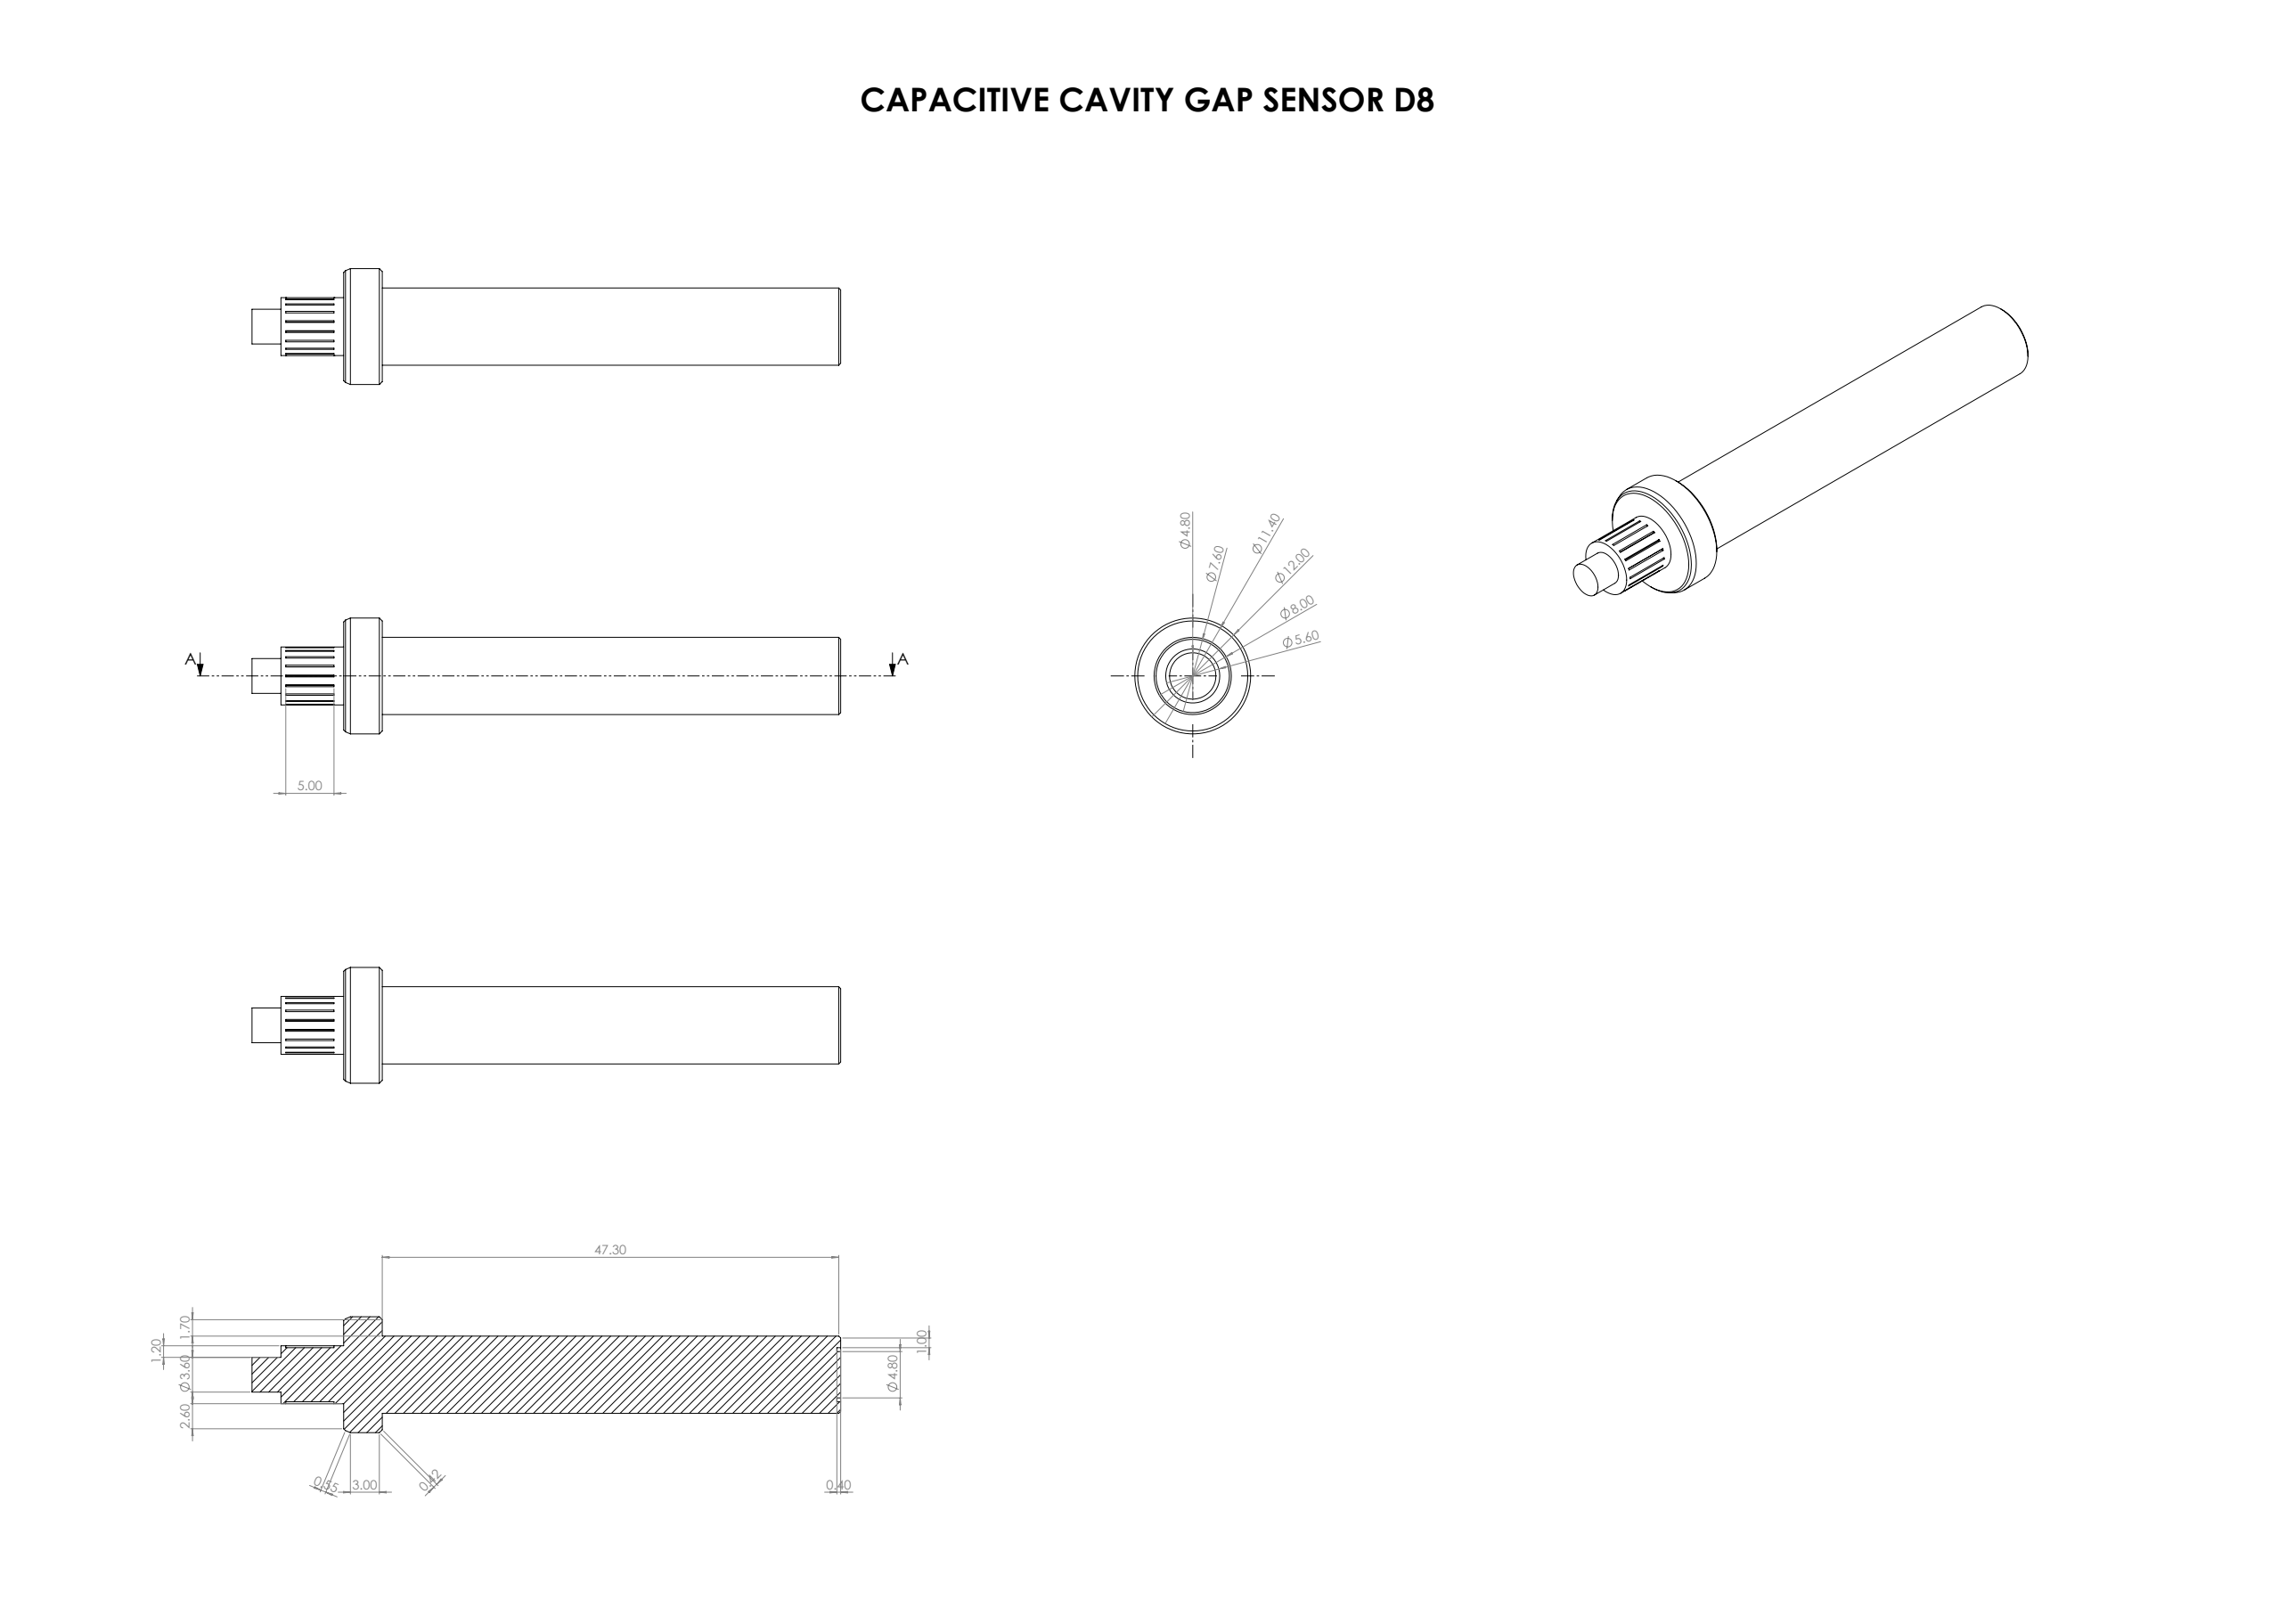
ISO-10303-21;
HEADER;
/* Generated by software containing ST-Developer
 * from STEP Tools, Inc. (www.steptools.com) 
 */

FILE_DESCRIPTION(
/* description */ (''),
/* implementation_level */ '2;1');

FILE_NAME(
/* name */ '07_Capacitive_Cavity_Gap_Sensor_D8.step',
/* time_stamp */ '2026-10-19T22:59:19-07:00',
/* author */ (''),
/* organization */ (''),
/* preprocessor_version */ 'ST-DEVELOPER v20.2',
/* originating_system */ 'Autodesk Translation Framework v15.15.0.0',
/* authorisation */ '');

FILE_SCHEMA (('AUTOMOTIVE_DESIGN { 1 0 10303 214 3 1 1 }'));
ENDSEC;

DATA;
#10=MECHANICAL_DESIGN_GEOMETRIC_PRESENTATION_REPRESENTATION('',(#919),#53650);
#887=SHAPE_REPRESENTATION_RELATIONSHIP('SRR','None',#53732,#903);
#903=ADVANCED_BREP_SHAPE_REPRESENTATION('',(#935),#53642);
#919=STYLED_ITEM('',(#53944),#935);
#935=MANIFOLD_SOLID_BREP('Gap Sensor',#23311);
#1038=CYLINDRICAL_SURFACE('',#24380,0.6);
#1039=CYLINDRICAL_SURFACE('',#24499,0.24);
#1040=CYLINDRICAL_SURFACE('',#24502,0.28);
#1041=CYLINDRICAL_SURFACE('',#24511,0.4);
#1042=CYLINDRICAL_SURFACE('',#24514,0.3);
#1043=CYLINDRICAL_SURFACE('',#24518,0.18);
#1388=FACE_BOUND('',#4169,.T.);
#1389=FACE_BOUND('',#4245,.T.);
#1390=FACE_BOUND('',#4247,.T.);
#1391=FACE_BOUND('',#4252,.T.);
#1392=FACE_BOUND('',#4254,.T.);
#1393=FACE_BOUND('',#4255,.T.);
#1394=FACE_BOUND('',#4256,.T.);
#1395=FACE_BOUND('',#4257,.T.);
#1396=FACE_BOUND('',#4258,.T.);
#1397=FACE_BOUND('',#4259,.T.);
#1398=FACE_BOUND('',#4260,.T.);
#1399=FACE_BOUND('',#4261,.T.);
#1400=FACE_BOUND('',#4262,.T.);
#1401=FACE_BOUND('',#4263,.T.);
#1402=FACE_BOUND('',#4264,.T.);
#1403=FACE_BOUND('',#4265,.T.);
#1404=FACE_BOUND('',#4266,.T.);
#1405=FACE_BOUND('',#4267,.T.);
#1406=FACE_BOUND('',#4268,.T.);
#1407=FACE_BOUND('',#4269,.T.);
#1408=FACE_BOUND('',#4270,.T.);
#1409=FACE_BOUND('',#4272,.T.);
#1676=PLANE('',#24387);
#1677=PLANE('',#24389);
#1678=PLANE('',#24390);
#1679=PLANE('',#24392);
#1680=PLANE('',#24393);
#1681=PLANE('',#24395);
#1682=PLANE('',#24396);
#1683=PLANE('',#24398);
#1684=PLANE('',#24399);
#1685=PLANE('',#24401);
#1686=PLANE('',#24402);
#1687=PLANE('',#24404);
#1688=PLANE('',#24405);
#1689=PLANE('',#24407);
#1690=PLANE('',#24408);
#1691=PLANE('',#24410);
#1692=PLANE('',#24411);
#1693=PLANE('',#24413);
#1694=PLANE('',#24414);
#1695=PLANE('',#24416);
#1696=PLANE('',#24417);
#1697=PLANE('',#24419);
#1698=PLANE('',#24420);
#1699=PLANE('',#24422);
#1700=PLANE('',#24423);
#1701=PLANE('',#24425);
#1702=PLANE('',#24426);
#1703=PLANE('',#24428);
#1704=PLANE('',#24429);
#1705=PLANE('',#24431);
#1706=PLANE('',#24432);
#1707=PLANE('',#24434);
#1708=PLANE('',#24435);
#1709=PLANE('',#24437);
#1710=PLANE('',#24438);
#1711=PLANE('',#24441);
#1712=PLANE('',#24442);
#1713=PLANE('',#24445);
#1714=PLANE('',#24446);
#1715=PLANE('',#24448);
#1716=PLANE('',#24449);
#1717=PLANE('',#24451);
#1718=PLANE('',#24452);
#1719=PLANE('',#24454);
#1720=PLANE('',#24455);
#1721=PLANE('',#24457);
#1722=PLANE('',#24458);
#1723=PLANE('',#24460);
#1724=PLANE('',#24461);
#1725=PLANE('',#24463);
#1726=PLANE('',#24464);
#1727=PLANE('',#24466);
#1728=PLANE('',#24467);
#1729=PLANE('',#24469);
#1730=PLANE('',#24470);
#1731=PLANE('',#24472);
#1732=PLANE('',#24473);
#1733=PLANE('',#24475);
#1734=PLANE('',#24476);
#1735=PLANE('',#24478);
#1736=PLANE('',#24479);
#1737=PLANE('',#24481);
#1738=PLANE('',#24482);
#1739=PLANE('',#24484);
#1740=PLANE('',#24485);
#1741=PLANE('',#24487);
#1742=PLANE('',#24488);
#1743=PLANE('',#24490);
#1744=PLANE('',#24491);
#1745=PLANE('',#24493);
#1746=PLANE('',#24494);
#1747=PLANE('',#24496);
#1748=PLANE('',#24497);
#1749=PLANE('',#24505);
#1750=PLANE('',#24506);
#1751=PLANE('',#24508);
#1752=PLANE('',#24512);
#1753=PLANE('',#24516);
#1754=PLANE('',#24520);
#2725=FACE_OUTER_BOUND('',#4164,.T.);
#2726=FACE_OUTER_BOUND('',#4165,.T.);
#2727=FACE_OUTER_BOUND('',#4166,.T.);
#2728=FACE_OUTER_BOUND('',#4167,.T.);
#2729=FACE_OUTER_BOUND('',#4168,.T.);
#2730=FACE_OUTER_BOUND('',#4170,.T.);
#2731=FACE_OUTER_BOUND('',#4171,.T.);
#2732=FACE_OUTER_BOUND('',#4172,.T.);
#2733=FACE_OUTER_BOUND('',#4173,.T.);
#2734=FACE_OUTER_BOUND('',#4174,.T.);
#2735=FACE_OUTER_BOUND('',#4175,.T.);
#2736=FACE_OUTER_BOUND('',#4176,.T.);
#2737=FACE_OUTER_BOUND('',#4177,.T.);
#2738=FACE_OUTER_BOUND('',#4178,.T.);
#2739=FACE_OUTER_BOUND('',#4179,.T.);
#2740=FACE_OUTER_BOUND('',#4180,.T.);
#2741=FACE_OUTER_BOUND('',#4181,.T.);
#2742=FACE_OUTER_BOUND('',#4182,.T.);
#2743=FACE_OUTER_BOUND('',#4183,.T.);
#2744=FACE_OUTER_BOUND('',#4184,.T.);
#2745=FACE_OUTER_BOUND('',#4185,.T.);
#2746=FACE_OUTER_BOUND('',#4186,.T.);
#2747=FACE_OUTER_BOUND('',#4187,.T.);
#2748=FACE_OUTER_BOUND('',#4188,.T.);
#2749=FACE_OUTER_BOUND('',#4189,.T.);
#2750=FACE_OUTER_BOUND('',#4190,.T.);
#2751=FACE_OUTER_BOUND('',#4191,.T.);
#2752=FACE_OUTER_BOUND('',#4192,.T.);
#2753=FACE_OUTER_BOUND('',#4193,.T.);
#2754=FACE_OUTER_BOUND('',#4194,.T.);
#2755=FACE_OUTER_BOUND('',#4195,.T.);
#2756=FACE_OUTER_BOUND('',#4196,.T.);
#2757=FACE_OUTER_BOUND('',#4197,.T.);
#2758=FACE_OUTER_BOUND('',#4198,.T.);
#2759=FACE_OUTER_BOUND('',#4199,.T.);
#2760=FACE_OUTER_BOUND('',#4200,.T.);
#2761=FACE_OUTER_BOUND('',#4201,.T.);
#2762=FACE_OUTER_BOUND('',#4202,.T.);
#2763=FACE_OUTER_BOUND('',#4203,.T.);
#2764=FACE_OUTER_BOUND('',#4204,.T.);
#2765=FACE_OUTER_BOUND('',#4205,.T.);
#2766=FACE_OUTER_BOUND('',#4206,.T.);
#2767=FACE_OUTER_BOUND('',#4207,.T.);
#2768=FACE_OUTER_BOUND('',#4208,.T.);
#2769=FACE_OUTER_BOUND('',#4209,.T.);
#2770=FACE_OUTER_BOUND('',#4210,.T.);
#2771=FACE_OUTER_BOUND('',#4211,.T.);
#2772=FACE_OUTER_BOUND('',#4212,.T.);
#2773=FACE_OUTER_BOUND('',#4213,.T.);
#2774=FACE_OUTER_BOUND('',#4214,.T.);
#2775=FACE_OUTER_BOUND('',#4215,.T.);
#2776=FACE_OUTER_BOUND('',#4216,.T.);
#2777=FACE_OUTER_BOUND('',#4217,.T.);
#2778=FACE_OUTER_BOUND('',#4218,.T.);
#2779=FACE_OUTER_BOUND('',#4219,.T.);
#2780=FACE_OUTER_BOUND('',#4220,.T.);
#2781=FACE_OUTER_BOUND('',#4221,.T.);
#2782=FACE_OUTER_BOUND('',#4222,.T.);
#2783=FACE_OUTER_BOUND('',#4223,.T.);
#2784=FACE_OUTER_BOUND('',#4224,.T.);
#2785=FACE_OUTER_BOUND('',#4225,.T.);
#2786=FACE_OUTER_BOUND('',#4226,.T.);
#2787=FACE_OUTER_BOUND('',#4227,.T.);
#2788=FACE_OUTER_BOUND('',#4228,.T.);
#2789=FACE_OUTER_BOUND('',#4229,.T.);
#2790=FACE_OUTER_BOUND('',#4230,.T.);
#2791=FACE_OUTER_BOUND('',#4231,.T.);
#2792=FACE_OUTER_BOUND('',#4232,.T.);
#2793=FACE_OUTER_BOUND('',#4233,.T.);
#2794=FACE_OUTER_BOUND('',#4234,.T.);
#2795=FACE_OUTER_BOUND('',#4235,.T.);
#2796=FACE_OUTER_BOUND('',#4236,.T.);
#2797=FACE_OUTER_BOUND('',#4237,.T.);
#2798=FACE_OUTER_BOUND('',#4238,.T.);
#2799=FACE_OUTER_BOUND('',#4239,.T.);
#2800=FACE_OUTER_BOUND('',#4240,.T.);
#2801=FACE_OUTER_BOUND('',#4241,.T.);
#2802=FACE_OUTER_BOUND('',#4242,.T.);
#2803=FACE_OUTER_BOUND('',#4243,.T.);
#2804=FACE_OUTER_BOUND('',#4244,.T.);
#2805=FACE_OUTER_BOUND('',#4246,.T.);
#2806=FACE_OUTER_BOUND('',#4248,.T.);
#2807=FACE_OUTER_BOUND('',#4249,.T.);
#2808=FACE_OUTER_BOUND('',#4250,.T.);
#2809=FACE_OUTER_BOUND('',#4251,.T.);
#2810=FACE_OUTER_BOUND('',#4253,.T.);
#2811=FACE_OUTER_BOUND('',#4271,.T.);
#2812=FACE_OUTER_BOUND('',#4273,.T.);
#2813=FACE_OUTER_BOUND('',#4274,.T.);
#4164=EDGE_LOOP('',(#17227,#17228,#17229,#17230,#17231,#17232));
#4165=EDGE_LOOP('',(#17233,#17234,#17235,#17236,#17237,#17238));
#4166=EDGE_LOOP('',(#17239,#17240,#17241,#17242,#17243));
#4167=EDGE_LOOP('',(#17244,#17245,#17246,#17247,#17248));
#4168=EDGE_LOOP('',(#17249));
#4169=EDGE_LOOP('',(#17250));
#4170=EDGE_LOOP('',(#17251,#17252,#17253,#17254));
#4171=EDGE_LOOP('',(#17255,#17256,#17257));
#4172=EDGE_LOOP('',(#17258,#17259,#17260,#17261));
#4173=EDGE_LOOP('',(#17262,#17263,#17264));
#4174=EDGE_LOOP('',(#17265,#17266,#17267,#17268));
#4175=EDGE_LOOP('',(#17269,#17270,#17271));
#4176=EDGE_LOOP('',(#17272,#17273,#17274,#17275));
#4177=EDGE_LOOP('',(#17276,#17277,#17278));
#4178=EDGE_LOOP('',(#17279,#17280,#17281,#17282));
#4179=EDGE_LOOP('',(#17283,#17284,#17285));
#4180=EDGE_LOOP('',(#17286,#17287,#17288,#17289));
#4181=EDGE_LOOP('',(#17290,#17291,#17292));
#4182=EDGE_LOOP('',(#17293,#17294,#17295,#17296));
#4183=EDGE_LOOP('',(#17297,#17298,#17299));
#4184=EDGE_LOOP('',(#17300,#17301,#17302,#17303));
#4185=EDGE_LOOP('',(#17304,#17305,#17306));
#4186=EDGE_LOOP('',(#17307,#17308,#17309,#17310));
#4187=EDGE_LOOP('',(#17311,#17312,#17313));
#4188=EDGE_LOOP('',(#17314,#17315,#17316,#17317));
#4189=EDGE_LOOP('',(#17318,#17319,#17320));
#4190=EDGE_LOOP('',(#17321,#17322,#17323,#17324));
#4191=EDGE_LOOP('',(#17325,#17326,#17327));
#4192=EDGE_LOOP('',(#17328,#17329,#17330,#17331));
#4193=EDGE_LOOP('',(#17332,#17333,#17334));
#4194=EDGE_LOOP('',(#17335,#17336,#17337,#17338));
#4195=EDGE_LOOP('',(#17339,#17340,#17341));
#4196=EDGE_LOOP('',(#17342,#17343,#17344,#17345));
#4197=EDGE_LOOP('',(#17346,#17347,#17348));
#4198=EDGE_LOOP('',(#17349,#17350,#17351,#17352));
#4199=EDGE_LOOP('',(#17353,#17354,#17355));
#4200=EDGE_LOOP('',(#17356,#17357,#17358,#17359));
#4201=EDGE_LOOP('',(#17360,#17361,#17362));
#4202=EDGE_LOOP('',(#17363,#17364,#17365,#17366));
#4203=EDGE_LOOP('',(#17367,#17368,#17369,#17370));
#4204=EDGE_LOOP('',(#17371,#17372,#17373,#17374));
#4205=EDGE_LOOP('',(#17375,#17376,#17377,#17378));
#4206=EDGE_LOOP('',(#17379,#17380,#17381,#17382));
#4207=EDGE_LOOP('',(#17383,#17384,#17385));
#4208=EDGE_LOOP('',(#17386,#17387,#17388,#17389));
#4209=EDGE_LOOP('',(#17390,#17391,#17392));
#4210=EDGE_LOOP('',(#17393,#17394,#17395,#17396));
#4211=EDGE_LOOP('',(#17397,#17398,#17399));
#4212=EDGE_LOOP('',(#17400,#17401,#17402,#17403));
#4213=EDGE_LOOP('',(#17404,#17405,#17406));
#4214=EDGE_LOOP('',(#17407,#17408,#17409,#17410));
#4215=EDGE_LOOP('',(#17411,#17412,#17413));
#4216=EDGE_LOOP('',(#17414,#17415,#17416,#17417));
#4217=EDGE_LOOP('',(#17418,#17419,#17420));
#4218=EDGE_LOOP('',(#17421,#17422,#17423,#17424));
#4219=EDGE_LOOP('',(#17425,#17426,#17427));
#4220=EDGE_LOOP('',(#17428,#17429,#17430,#17431));
#4221=EDGE_LOOP('',(#17432,#17433,#17434));
#4222=EDGE_LOOP('',(#17435,#17436,#17437,#17438));
#4223=EDGE_LOOP('',(#17439,#17440,#17441));
#4224=EDGE_LOOP('',(#17442,#17443,#17444,#17445));
#4225=EDGE_LOOP('',(#17446,#17447,#17448));
#4226=EDGE_LOOP('',(#17449,#17450,#17451,#17452));
#4227=EDGE_LOOP('',(#17453,#17454,#17455));
#4228=EDGE_LOOP('',(#17456,#17457,#17458,#17459));
#4229=EDGE_LOOP('',(#17460,#17461,#17462));
#4230=EDGE_LOOP('',(#17463,#17464,#17465,#17466));
#4231=EDGE_LOOP('',(#17467,#17468,#17469));
#4232=EDGE_LOOP('',(#17470,#17471,#17472,#17473));
#4233=EDGE_LOOP('',(#17474,#17475,#17476));
#4234=EDGE_LOOP('',(#17477,#17478,#17479,#17480));
#4235=EDGE_LOOP('',(#17481,#17482,#17483));
#4236=EDGE_LOOP('',(#17484,#17485,#17486,#17487));
#4237=EDGE_LOOP('',(#17488,#17489,#17490));
#4238=EDGE_LOOP('',(#17491,#17492,#17493,#17494));
#4239=EDGE_LOOP('',(#17495,#17496,#17497));
#4240=EDGE_LOOP('',(#17498,#17499,#17500,#17501));
#4241=EDGE_LOOP('',(#17502,#17503,#17504));
#4242=EDGE_LOOP('',(#17505,#17506,#17507,#17508));
#4243=EDGE_LOOP('',(#17509,#17510,#17511,#17512));
#4244=EDGE_LOOP('',(#17513));
#4245=EDGE_LOOP('',(#17514));
#4246=EDGE_LOOP('',(#17515));
#4247=EDGE_LOOP('',(#17516));
#4248=EDGE_LOOP('',(#17517));
#4249=EDGE_LOOP('',(#17518,#17519,#17520,#17521));
#4250=EDGE_LOOP('',(#17522,#17523,#17524,#17525));
#4251=EDGE_LOOP('',(#17526));
#4252=EDGE_LOOP('',(#17527));
#4253=EDGE_LOOP('',(#17528,#17529,#17530,#17531,#17532,#17533,#17534,#17535,
#17536,#17537,#17538,#17539));
#4254=EDGE_LOOP('',(#17540,#17541,#17542,#17543));
#4255=EDGE_LOOP('',(#17544,#17545,#17546,#17547));
#4256=EDGE_LOOP('',(#17548,#17549,#17550,#17551));
#4257=EDGE_LOOP('',(#17552,#17553,#17554,#17555));
#4258=EDGE_LOOP('',(#17556,#17557,#17558,#17559));
#4259=EDGE_LOOP('',(#17560,#17561,#17562,#17563));
#4260=EDGE_LOOP('',(#17564,#17565,#17566,#17567));
#4261=EDGE_LOOP('',(#17568,#17569,#17570,#17571));
#4262=EDGE_LOOP('',(#17572,#17573,#17574,#17575));
#4263=EDGE_LOOP('',(#17576,#17577,#17578,#17579));
#4264=EDGE_LOOP('',(#17580,#17581,#17582,#17583));
#4265=EDGE_LOOP('',(#17584,#17585,#17586,#17587));
#4266=EDGE_LOOP('',(#17588,#17589,#17590,#17591));
#4267=EDGE_LOOP('',(#17592,#17593,#17594,#17595));
#4268=EDGE_LOOP('',(#17596,#17597,#17598,#17599));
#4269=EDGE_LOOP('',(#17600,#17601,#17602,#17603));
#4270=EDGE_LOOP('',(#17604,#17605,#17606,#17607));
#4271=EDGE_LOOP('',(#17608));
#4272=EDGE_LOOP('',(#17609));
#4273=EDGE_LOOP('',(#17610,#17611,#17612,#17613));
#4274=EDGE_LOOP('',(#17614));
#5445=CIRCLE('',#24376,0.578786796564404);
#5446=CIRCLE('',#24377,0.578786796564404);
#5447=CIRCLE('',#24378,0.6);
#5448=CIRCLE('',#24379,0.6);
#5449=CIRCLE('',#24381,0.6);
#5450=CIRCLE('',#24382,0.6);
#5451=CIRCLE('',#24384,0.56);
#5452=CIRCLE('',#24386,0.57);
#5453=CIRCLE('',#24388,0.4);
#5454=CIRCLE('',#24391,0.3);
#5455=CIRCLE('',#24394,0.3);
#5456=CIRCLE('',#24397,0.3);
#5457=CIRCLE('',#24400,0.3);
#5458=CIRCLE('',#24403,0.3);
#5459=CIRCLE('',#24406,0.3);
#5460=CIRCLE('',#24409,0.3);
#5461=CIRCLE('',#24412,0.3);
#5462=CIRCLE('',#24415,0.3);
#5463=CIRCLE('',#24418,0.3);
#5464=CIRCLE('',#24421,0.3);
#5465=CIRCLE('',#24424,0.3);
#5466=CIRCLE('',#24427,0.3);
#5467=CIRCLE('',#24430,0.3);
#5468=CIRCLE('',#24433,0.3);
#5469=CIRCLE('',#24436,0.3);
#5470=CIRCLE('',#24439,0.3);
#5471=CIRCLE('',#24440,0.3);
#5472=CIRCLE('',#24443,0.3);
#5473=CIRCLE('',#24444,0.3);
#5474=CIRCLE('',#24447,0.3);
#5475=CIRCLE('',#24450,0.3);
#5476=CIRCLE('',#24453,0.3);
#5477=CIRCLE('',#24456,0.3);
#5478=CIRCLE('',#24459,0.3);
#5479=CIRCLE('',#24462,0.3);
#5480=CIRCLE('',#24465,0.3);
#5481=CIRCLE('',#24468,0.3);
#5482=CIRCLE('',#24471,0.3);
#5483=CIRCLE('',#24474,0.3);
#5484=CIRCLE('',#24477,0.3);
#5485=CIRCLE('',#24480,0.3);
#5486=CIRCLE('',#24483,0.3);
#5487=CIRCLE('',#24486,0.3);
#5488=CIRCLE('',#24489,0.3);
#5489=CIRCLE('',#24492,0.3);
#5490=CIRCLE('',#24495,0.3);
#5491=CIRCLE('',#24498,0.3);
#5492=CIRCLE('',#24500,0.24);
#5493=CIRCLE('',#24501,0.24);
#5494=CIRCLE('',#24503,0.28);
#5495=CIRCLE('',#24504,0.28);
#5496=CIRCLE('',#24507,0.38);
#5497=CIRCLE('',#24510,0.4);
#5498=CIRCLE('',#24513,0.3);
#5499=CIRCLE('',#24515,0.3);
#5500=CIRCLE('',#24517,0.18);
#5501=CIRCLE('',#24519,0.18);
#6499=LINE('',#35561,#8344);
#6500=LINE('',#35567,#8345);
#6501=LINE('',#35574,#8346);
#6502=LINE('',#35577,#8347);
#6503=LINE('',#35585,#8348);
#6504=LINE('',#35587,#8349);
#6505=LINE('',#35589,#8350);
#6506=LINE('',#35590,#8351);
#6507=LINE('',#35594,#8352);
#6508=LINE('',#35597,#8353);
#6509=LINE('',#35598,#8354);
#6510=LINE('',#35604,#8355);
#6511=LINE('',#35606,#8356);
#6512=LINE('',#35608,#8357);
#6513=LINE('',#35609,#8358);
#6514=LINE('',#35613,#8359);
#6515=LINE('',#35616,#8360);
#6516=LINE('',#35617,#8361);
#6517=LINE('',#35623,#8362);
#6518=LINE('',#35625,#8363);
#6519=LINE('',#35627,#8364);
#6520=LINE('',#35628,#8365);
#6521=LINE('',#35632,#8366);
#6522=LINE('',#35635,#8367);
#6523=LINE('',#35636,#8368);
#6524=LINE('',#35642,#8369);
#6525=LINE('',#35644,#8370);
#6526=LINE('',#35646,#8371);
#6527=LINE('',#35647,#8372);
#6528=LINE('',#35651,#8373);
#6529=LINE('',#35654,#8374);
#6530=LINE('',#35655,#8375);
#6531=LINE('',#35661,#8376);
#6532=LINE('',#35663,#8377);
#6533=LINE('',#35665,#8378);
#6534=LINE('',#35666,#8379);
#6535=LINE('',#35670,#8380);
#6536=LINE('',#35673,#8381);
#6537=LINE('',#35674,#8382);
#6538=LINE('',#35680,#8383);
#6539=LINE('',#35682,#8384);
#6540=LINE('',#35684,#8385);
#6541=LINE('',#35685,#8386);
#6542=LINE('',#35689,#8387);
#6543=LINE('',#35692,#8388);
#6544=LINE('',#35693,#8389);
#6545=LINE('',#35699,#8390);
#6546=LINE('',#35701,#8391);
#6547=LINE('',#35703,#8392);
#6548=LINE('',#35704,#8393);
#6549=LINE('',#35708,#8394);
#6550=LINE('',#35711,#8395);
#6551=LINE('',#35712,#8396);
#6552=LINE('',#35718,#8397);
#6553=LINE('',#35720,#8398);
#6554=LINE('',#35722,#8399);
#6555=LINE('',#35723,#8400);
#6556=LINE('',#35727,#8401);
#6557=LINE('',#35730,#8402);
#6558=LINE('',#35731,#8403);
#6559=LINE('',#35737,#8404);
#6560=LINE('',#35739,#8405);
#6561=LINE('',#35741,#8406);
#6562=LINE('',#35742,#8407);
#6563=LINE('',#35747,#8408);
#6564=LINE('',#35751,#8409);
#6565=LINE('',#35752,#8410);
#6566=LINE('',#35760,#8411);
#6567=LINE('',#35762,#8412);
#6568=LINE('',#35764,#8413);
#6569=LINE('',#35765,#8414);
#6570=LINE('',#35769,#8415);
#6571=LINE('',#35772,#8416);
#6572=LINE('',#35773,#8417);
#6573=LINE('',#35779,#8418);
#6574=LINE('',#35781,#8419);
#6575=LINE('',#35783,#8420);
#6576=LINE('',#35784,#8421);
#6577=LINE('',#35788,#8422);
#6578=LINE('',#35791,#8423);
#6579=LINE('',#35792,#8424);
#6580=LINE('',#35798,#8425);
#6581=LINE('',#35800,#8426);
#6582=LINE('',#35802,#8427);
#6583=LINE('',#35803,#8428);
#6584=LINE('',#35807,#8429);
#6585=LINE('',#35810,#8430);
#6586=LINE('',#35811,#8431);
#6587=LINE('',#35817,#8432);
#6588=LINE('',#35819,#8433);
#6589=LINE('',#35821,#8434);
#6590=LINE('',#35822,#8435);
#6591=LINE('',#35826,#8436);
#6592=LINE('',#35829,#8437);
#6593=LINE('',#35830,#8438);
#6594=LINE('',#35836,#8439);
#6595=LINE('',#35838,#8440);
#6596=LINE('',#35840,#8441);
#6597=LINE('',#35841,#8442);
#6598=LINE('',#35845,#8443);
#6599=LINE('',#35848,#8444);
#6600=LINE('',#35849,#8445);
#6601=LINE('',#35855,#8446);
#6602=LINE('',#35857,#8447);
#6603=LINE('',#35859,#8448);
#6604=LINE('',#35860,#8449);
#6605=LINE('',#35864,#8450);
#6606=LINE('',#35867,#8451);
#6607=LINE('',#35868,#8452);
#6608=LINE('',#35874,#8453);
#6609=LINE('',#35876,#8454);
#6610=LINE('',#35878,#8455);
#6611=LINE('',#35879,#8456);
#6612=LINE('',#35883,#8457);
#6613=LINE('',#35886,#8458);
#6614=LINE('',#35887,#8459);
#6615=LINE('',#35893,#8460);
#6616=LINE('',#35895,#8461);
#6617=LINE('',#35897,#8462);
#6618=LINE('',#35898,#8463);
#6619=LINE('',#35902,#8464);
#6620=LINE('',#35905,#8465);
#6621=LINE('',#35906,#8466);
#6622=LINE('',#35912,#8467);
#6623=LINE('',#35914,#8468);
#6624=LINE('',#35916,#8469);
#6625=LINE('',#35917,#8470);
#6626=LINE('',#35921,#8471);
#6627=LINE('',#35924,#8472);
#6628=LINE('',#35925,#8473);
#6629=LINE('',#35932,#8474);
#6630=LINE('',#35938,#8475);
#6631=LINE('',#35948,#8476);
#6632=LINE('',#35950,#8477);
#6633=LINE('',#35957,#8478);
#6634=LINE('',#35958,#8479);
#6635=LINE('',#35965,#8480);
#8344=VECTOR('',#28065,0.589393398282202);
#8345=VECTOR('',#28072,0.6);
#8346=VECTOR('',#28081,0.58);
#8347=VECTOR('',#28084,0.585);
#8348=VECTOR('',#28093,1.);
#8349=VECTOR('',#28094,1.);
#8350=VECTOR('',#28095,1.);
#8351=VECTOR('',#28096,1.);
#8352=VECTOR('',#28101,1.);
#8353=VECTOR('',#28104,1.);
#8354=VECTOR('',#28105,1.);
#8355=VECTOR('',#28112,1.);
#8356=VECTOR('',#28113,1.);
#8357=VECTOR('',#28114,1.);
#8358=VECTOR('',#28115,1.);
#8359=VECTOR('',#28120,1.);
#8360=VECTOR('',#28123,1.);
#8361=VECTOR('',#28124,1.);
#8362=VECTOR('',#28131,1.);
#8363=VECTOR('',#28132,1.);
#8364=VECTOR('',#28133,1.);
#8365=VECTOR('',#28134,1.);
#8366=VECTOR('',#28139,1.);
#8367=VECTOR('',#28142,1.);
#8368=VECTOR('',#28143,1.);
#8369=VECTOR('',#28150,1.);
#8370=VECTOR('',#28151,1.);
#8371=VECTOR('',#28152,1.);
#8372=VECTOR('',#28153,1.);
#8373=VECTOR('',#28158,1.);
#8374=VECTOR('',#28161,1.);
#8375=VECTOR('',#28162,1.);
#8376=VECTOR('',#28169,1.);
#8377=VECTOR('',#28170,1.);
#8378=VECTOR('',#28171,1.);
#8379=VECTOR('',#28172,1.);
#8380=VECTOR('',#28177,1.);
#8381=VECTOR('',#28180,1.);
#8382=VECTOR('',#28181,1.);
#8383=VECTOR('',#28188,1.);
#8384=VECTOR('',#28189,1.);
#8385=VECTOR('',#28190,1.);
#8386=VECTOR('',#28191,1.);
#8387=VECTOR('',#28196,1.);
#8388=VECTOR('',#28199,1.);
#8389=VECTOR('',#28200,1.);
#8390=VECTOR('',#28207,1.);
#8391=VECTOR('',#28208,1.);
#8392=VECTOR('',#28209,1.);
#8393=VECTOR('',#28210,1.);
#8394=VECTOR('',#28215,1.);
#8395=VECTOR('',#28218,1.);
#8396=VECTOR('',#28219,1.);
#8397=VECTOR('',#28226,1.);
#8398=VECTOR('',#28227,1.);
#8399=VECTOR('',#28228,1.);
#8400=VECTOR('',#28229,1.);
#8401=VECTOR('',#28234,1.);
#8402=VECTOR('',#28237,1.);
#8403=VECTOR('',#28238,1.);
#8404=VECTOR('',#28245,1.);
#8405=VECTOR('',#28246,1.);
#8406=VECTOR('',#28247,1.);
#8407=VECTOR('',#28248,1.);
#8408=VECTOR('',#28253,1.);
#8409=VECTOR('',#28258,1.);
#8410=VECTOR('',#28259,1.);
#8411=VECTOR('',#28268,1.);
#8412=VECTOR('',#28269,1.);
#8413=VECTOR('',#28270,1.);
#8414=VECTOR('',#28271,1.);
#8415=VECTOR('',#28276,1.);
#8416=VECTOR('',#28279,1.);
#8417=VECTOR('',#28280,1.);
#8418=VECTOR('',#28287,1.);
#8419=VECTOR('',#28288,1.);
#8420=VECTOR('',#28289,1.);
#8421=VECTOR('',#28290,1.);
#8422=VECTOR('',#28295,1.);
#8423=VECTOR('',#28298,1.);
#8424=VECTOR('',#28299,1.);
#8425=VECTOR('',#28306,1.);
#8426=VECTOR('',#28307,1.);
#8427=VECTOR('',#28308,1.);
#8428=VECTOR('',#28309,1.);
#8429=VECTOR('',#28314,1.);
#8430=VECTOR('',#28317,1.);
#8431=VECTOR('',#28318,1.);
#8432=VECTOR('',#28325,1.);
#8433=VECTOR('',#28326,1.);
#8434=VECTOR('',#28327,1.);
#8435=VECTOR('',#28328,1.);
#8436=VECTOR('',#28333,1.);
#8437=VECTOR('',#28336,1.);
#8438=VECTOR('',#28337,1.);
#8439=VECTOR('',#28344,1.);
#8440=VECTOR('',#28345,1.);
#8441=VECTOR('',#28346,1.);
#8442=VECTOR('',#28347,1.);
#8443=VECTOR('',#28352,1.);
#8444=VECTOR('',#28355,1.);
#8445=VECTOR('',#28356,1.);
#8446=VECTOR('',#28363,1.);
#8447=VECTOR('',#28364,1.);
#8448=VECTOR('',#28365,1.);
#8449=VECTOR('',#28366,1.);
#8450=VECTOR('',#28371,1.);
#8451=VECTOR('',#28374,1.);
#8452=VECTOR('',#28375,1.);
#8453=VECTOR('',#28382,1.);
#8454=VECTOR('',#28383,1.);
#8455=VECTOR('',#28384,1.);
#8456=VECTOR('',#28385,1.);
#8457=VECTOR('',#28390,1.);
#8458=VECTOR('',#28393,1.);
#8459=VECTOR('',#28394,1.);
#8460=VECTOR('',#28401,1.);
#8461=VECTOR('',#28402,1.);
#8462=VECTOR('',#28403,1.);
#8463=VECTOR('',#28404,1.);
#8464=VECTOR('',#28409,1.);
#8465=VECTOR('',#28412,1.);
#8466=VECTOR('',#28413,1.);
#8467=VECTOR('',#28420,1.);
#8468=VECTOR('',#28421,1.);
#8469=VECTOR('',#28422,1.);
#8470=VECTOR('',#28423,1.);
#8471=VECTOR('',#28428,1.);
#8472=VECTOR('',#28431,1.);
#8473=VECTOR('',#28432,1.);
#8474=VECTOR('',#28441,0.24);
#8475=VECTOR('',#28448,0.28);
#8476=VECTOR('',#28463,0.39);
#8477=VECTOR('',#28466,0.4);
#8478=VECTOR('',#28475,0.3);
#8479=VECTOR('',#28476,0.3);
#8480=VECTOR('',#28485,0.18);
#10204=VERTEX_POINT('',#35556);
#10205=VERTEX_POINT('',#35557);
#10206=VERTEX_POINT('',#35560);
#10207=VERTEX_POINT('',#35562);
#10208=VERTEX_POINT('',#35566);
#10209=VERTEX_POINT('',#35568);
#10210=VERTEX_POINT('',#35572);
#10211=VERTEX_POINT('',#35576);
#10212=VERTEX_POINT('',#35580);
#10213=VERTEX_POINT('',#35583);
#10214=VERTEX_POINT('',#35584);
#10215=VERTEX_POINT('',#35586);
#10216=VERTEX_POINT('',#35588);
#10217=VERTEX_POINT('',#35592);
#10218=VERTEX_POINT('',#35596);
#10219=VERTEX_POINT('',#35602);
#10220=VERTEX_POINT('',#35603);
#10221=VERTEX_POINT('',#35605);
#10222=VERTEX_POINT('',#35607);
#10223=VERTEX_POINT('',#35611);
#10224=VERTEX_POINT('',#35615);
#10225=VERTEX_POINT('',#35621);
#10226=VERTEX_POINT('',#35622);
#10227=VERTEX_POINT('',#35624);
#10228=VERTEX_POINT('',#35626);
#10229=VERTEX_POINT('',#35630);
#10230=VERTEX_POINT('',#35634);
#10231=VERTEX_POINT('',#35640);
#10232=VERTEX_POINT('',#35641);
#10233=VERTEX_POINT('',#35643);
#10234=VERTEX_POINT('',#35645);
#10235=VERTEX_POINT('',#35649);
#10236=VERTEX_POINT('',#35653);
#10237=VERTEX_POINT('',#35659);
#10238=VERTEX_POINT('',#35660);
#10239=VERTEX_POINT('',#35662);
#10240=VERTEX_POINT('',#35664);
#10241=VERTEX_POINT('',#35668);
#10242=VERTEX_POINT('',#35672);
#10243=VERTEX_POINT('',#35678);
#10244=VERTEX_POINT('',#35679);
#10245=VERTEX_POINT('',#35681);
#10246=VERTEX_POINT('',#35683);
#10247=VERTEX_POINT('',#35687);
#10248=VERTEX_POINT('',#35691);
#10249=VERTEX_POINT('',#35697);
#10250=VERTEX_POINT('',#35698);
#10251=VERTEX_POINT('',#35700);
#10252=VERTEX_POINT('',#35702);
#10253=VERTEX_POINT('',#35706);
#10254=VERTEX_POINT('',#35710);
#10255=VERTEX_POINT('',#35716);
#10256=VERTEX_POINT('',#35717);
#10257=VERTEX_POINT('',#35719);
#10258=VERTEX_POINT('',#35721);
#10259=VERTEX_POINT('',#35725);
#10260=VERTEX_POINT('',#35729);
#10261=VERTEX_POINT('',#35735);
#10262=VERTEX_POINT('',#35736);
#10263=VERTEX_POINT('',#35738);
#10264=VERTEX_POINT('',#35740);
#10265=VERTEX_POINT('',#35744);
#10266=VERTEX_POINT('',#35746);
#10267=VERTEX_POINT('',#35750);
#10268=VERTEX_POINT('',#35754);
#10269=VERTEX_POINT('',#35758);
#10270=VERTEX_POINT('',#35759);
#10271=VERTEX_POINT('',#35761);
#10272=VERTEX_POINT('',#35763);
#10273=VERTEX_POINT('',#35767);
#10274=VERTEX_POINT('',#35771);
#10275=VERTEX_POINT('',#35777);
#10276=VERTEX_POINT('',#35778);
#10277=VERTEX_POINT('',#35780);
#10278=VERTEX_POINT('',#35782);
#10279=VERTEX_POINT('',#35786);
#10280=VERTEX_POINT('',#35790);
#10281=VERTEX_POINT('',#35796);
#10282=VERTEX_POINT('',#35797);
#10283=VERTEX_POINT('',#35799);
#10284=VERTEX_POINT('',#35801);
#10285=VERTEX_POINT('',#35805);
#10286=VERTEX_POINT('',#35809);
#10287=VERTEX_POINT('',#35815);
#10288=VERTEX_POINT('',#35816);
#10289=VERTEX_POINT('',#35818);
#10290=VERTEX_POINT('',#35820);
#10291=VERTEX_POINT('',#35824);
#10292=VERTEX_POINT('',#35828);
#10293=VERTEX_POINT('',#35834);
#10294=VERTEX_POINT('',#35835);
#10295=VERTEX_POINT('',#35837);
#10296=VERTEX_POINT('',#35839);
#10297=VERTEX_POINT('',#35843);
#10298=VERTEX_POINT('',#35847);
#10299=VERTEX_POINT('',#35853);
#10300=VERTEX_POINT('',#35854);
#10301=VERTEX_POINT('',#35856);
#10302=VERTEX_POINT('',#35858);
#10303=VERTEX_POINT('',#35862);
#10304=VERTEX_POINT('',#35866);
#10305=VERTEX_POINT('',#35872);
#10306=VERTEX_POINT('',#35873);
#10307=VERTEX_POINT('',#35875);
#10308=VERTEX_POINT('',#35877);
#10309=VERTEX_POINT('',#35881);
#10310=VERTEX_POINT('',#35885);
#10311=VERTEX_POINT('',#35891);
#10312=VERTEX_POINT('',#35892);
#10313=VERTEX_POINT('',#35894);
#10314=VERTEX_POINT('',#35896);
#10315=VERTEX_POINT('',#35900);
#10316=VERTEX_POINT('',#35904);
#10317=VERTEX_POINT('',#35910);
#10318=VERTEX_POINT('',#35911);
#10319=VERTEX_POINT('',#35913);
#10320=VERTEX_POINT('',#35915);
#10321=VERTEX_POINT('',#35919);
#10322=VERTEX_POINT('',#35923);
#10323=VERTEX_POINT('',#35929);
#10324=VERTEX_POINT('',#35931);
#10325=VERTEX_POINT('',#35935);
#10326=VERTEX_POINT('',#35937);
#10327=VERTEX_POINT('',#35942);
#10328=VERTEX_POINT('',#35946);
#10329=VERTEX_POINT('',#35952);
#10330=VERTEX_POINT('',#35955);
#10331=VERTEX_POINT('',#35960);
#10332=VERTEX_POINT('',#35963);
#12791=EDGE_CURVE('',#10204,#10205,#5445,.T.);
#12792=EDGE_CURVE('',#10205,#10204,#5446,.T.);
#12793=EDGE_CURVE('',#10204,#10206,#6499,.T.);
#12794=EDGE_CURVE('',#10206,#10207,#5447,.T.);
#12795=EDGE_CURVE('',#10207,#10206,#5448,.T.);
#12796=EDGE_CURVE('',#10207,#10208,#6500,.T.);
#12797=EDGE_CURVE('',#10209,#10208,#5449,.T.);
#12798=EDGE_CURVE('',#10208,#10209,#5450,.T.);
#12799=EDGE_CURVE('',#10210,#10210,#5451,.T.);
#12800=EDGE_CURVE('',#10210,#10205,#6501,.T.);
#12801=EDGE_CURVE('',#10209,#10211,#6502,.T.);
#12802=EDGE_CURVE('',#10211,#10211,#5452,.T.);
#12803=EDGE_CURVE('',#10212,#10212,#5453,.T.);
#12804=EDGE_CURVE('',#10213,#10214,#6503,.T.);
#12805=EDGE_CURVE('',#10215,#10213,#6504,.T.);
#12806=EDGE_CURVE('',#10215,#10216,#6505,.T.);
#12807=EDGE_CURVE('',#10216,#10214,#6506,.T.);
#12808=EDGE_CURVE('',#10214,#10217,#5454,.T.);
#12809=EDGE_CURVE('',#10217,#10216,#6507,.T.);
#12810=EDGE_CURVE('',#10217,#10218,#6508,.T.);
#12811=EDGE_CURVE('',#10218,#10215,#6509,.T.);
#12812=EDGE_CURVE('',#10218,#10213,#5455,.T.);
#12813=EDGE_CURVE('',#10219,#10220,#6510,.T.);
#12814=EDGE_CURVE('',#10221,#10219,#6511,.T.);
#12815=EDGE_CURVE('',#10221,#10222,#6512,.T.);
#12816=EDGE_CURVE('',#10222,#10220,#6513,.T.);
#12817=EDGE_CURVE('',#10220,#10223,#5456,.T.);
#12818=EDGE_CURVE('',#10223,#10222,#6514,.T.);
#12819=EDGE_CURVE('',#10223,#10224,#6515,.T.);
#12820=EDGE_CURVE('',#10224,#10221,#6516,.T.);
#12821=EDGE_CURVE('',#10224,#10219,#5457,.T.);
#12822=EDGE_CURVE('',#10225,#10226,#6517,.T.);
#12823=EDGE_CURVE('',#10227,#10225,#6518,.T.);
#12824=EDGE_CURVE('',#10227,#10228,#6519,.T.);
#12825=EDGE_CURVE('',#10228,#10226,#6520,.T.);
#12826=EDGE_CURVE('',#10226,#10229,#5458,.T.);
#12827=EDGE_CURVE('',#10229,#10228,#6521,.T.);
#12828=EDGE_CURVE('',#10229,#10230,#6522,.T.);
#12829=EDGE_CURVE('',#10230,#10227,#6523,.T.);
#12830=EDGE_CURVE('',#10230,#10225,#5459,.T.);
#12831=EDGE_CURVE('',#10231,#10232,#6524,.T.);
#12832=EDGE_CURVE('',#10233,#10231,#6525,.T.);
#12833=EDGE_CURVE('',#10233,#10234,#6526,.T.);
#12834=EDGE_CURVE('',#10234,#10232,#6527,.T.);
#12835=EDGE_CURVE('',#10232,#10235,#5460,.T.);
#12836=EDGE_CURVE('',#10235,#10234,#6528,.T.);
#12837=EDGE_CURVE('',#10235,#10236,#6529,.T.);
#12838=EDGE_CURVE('',#10236,#10233,#6530,.T.);
#12839=EDGE_CURVE('',#10236,#10231,#5461,.T.);
#12840=EDGE_CURVE('',#10237,#10238,#6531,.T.);
#12841=EDGE_CURVE('',#10239,#10237,#6532,.T.);
#12842=EDGE_CURVE('',#10239,#10240,#6533,.T.);
#12843=EDGE_CURVE('',#10240,#10238,#6534,.T.);
#12844=EDGE_CURVE('',#10238,#10241,#5462,.T.);
#12845=EDGE_CURVE('',#10241,#10240,#6535,.T.);
#12846=EDGE_CURVE('',#10241,#10242,#6536,.T.);
#12847=EDGE_CURVE('',#10242,#10239,#6537,.T.);
#12848=EDGE_CURVE('',#10242,#10237,#5463,.T.);
#12849=EDGE_CURVE('',#10243,#10244,#6538,.T.);
#12850=EDGE_CURVE('',#10245,#10243,#6539,.T.);
#12851=EDGE_CURVE('',#10245,#10246,#6540,.T.);
#12852=EDGE_CURVE('',#10246,#10244,#6541,.T.);
#12853=EDGE_CURVE('',#10244,#10247,#5464,.T.);
#12854=EDGE_CURVE('',#10247,#10246,#6542,.T.);
#12855=EDGE_CURVE('',#10247,#10248,#6543,.T.);
#12856=EDGE_CURVE('',#10248,#10245,#6544,.T.);
#12857=EDGE_CURVE('',#10248,#10243,#5465,.T.);
#12858=EDGE_CURVE('',#10249,#10250,#6545,.T.);
#12859=EDGE_CURVE('',#10251,#10249,#6546,.T.);
#12860=EDGE_CURVE('',#10251,#10252,#6547,.T.);
#12861=EDGE_CURVE('',#10252,#10250,#6548,.T.);
#12862=EDGE_CURVE('',#10250,#10253,#5466,.T.);
#12863=EDGE_CURVE('',#10253,#10252,#6549,.T.);
#12864=EDGE_CURVE('',#10253,#10254,#6550,.T.);
#12865=EDGE_CURVE('',#10254,#10251,#6551,.T.);
#12866=EDGE_CURVE('',#10254,#10249,#5467,.T.);
#12867=EDGE_CURVE('',#10255,#10256,#6552,.T.);
#12868=EDGE_CURVE('',#10257,#10255,#6553,.T.);
#12869=EDGE_CURVE('',#10257,#10258,#6554,.T.);
#12870=EDGE_CURVE('',#10258,#10256,#6555,.T.);
#12871=EDGE_CURVE('',#10256,#10259,#5468,.T.);
#12872=EDGE_CURVE('',#10259,#10258,#6556,.T.);
#12873=EDGE_CURVE('',#10259,#10260,#6557,.T.);
#12874=EDGE_CURVE('',#10260,#10257,#6558,.T.);
#12875=EDGE_CURVE('',#10260,#10255,#5469,.T.);
#12876=EDGE_CURVE('',#10261,#10262,#6559,.T.);
#12877=EDGE_CURVE('',#10263,#10261,#6560,.T.);
#12878=EDGE_CURVE('',#10263,#10264,#6561,.T.);
#12879=EDGE_CURVE('',#10264,#10262,#6562,.T.);
#12880=EDGE_CURVE('',#10262,#10265,#5470,.T.);
#12881=EDGE_CURVE('',#10266,#10264,#6563,.T.);
#12882=EDGE_CURVE('',#10265,#10266,#5471,.T.);
#12883=EDGE_CURVE('',#10266,#10267,#6564,.T.);
#12884=EDGE_CURVE('',#10267,#10263,#6565,.T.);
#12885=EDGE_CURVE('',#10267,#10268,#5472,.T.);
#12886=EDGE_CURVE('',#10268,#10261,#5473,.T.);
#12887=EDGE_CURVE('',#10269,#10270,#6566,.T.);
#12888=EDGE_CURVE('',#10271,#10269,#6567,.T.);
#12889=EDGE_CURVE('',#10271,#10272,#6568,.T.);
#12890=EDGE_CURVE('',#10272,#10270,#6569,.T.);
#12891=EDGE_CURVE('',#10270,#10273,#5474,.T.);
#12892=EDGE_CURVE('',#10273,#10272,#6570,.T.);
#12893=EDGE_CURVE('',#10273,#10274,#6571,.T.);
#12894=EDGE_CURVE('',#10274,#10271,#6572,.T.);
#12895=EDGE_CURVE('',#10274,#10269,#5475,.T.);
#12896=EDGE_CURVE('',#10275,#10276,#6573,.T.);
#12897=EDGE_CURVE('',#10277,#10275,#6574,.T.);
#12898=EDGE_CURVE('',#10277,#10278,#6575,.T.);
#12899=EDGE_CURVE('',#10278,#10276,#6576,.T.);
#12900=EDGE_CURVE('',#10276,#10279,#5476,.T.);
#12901=EDGE_CURVE('',#10279,#10278,#6577,.T.);
#12902=EDGE_CURVE('',#10279,#10280,#6578,.T.);
#12903=EDGE_CURVE('',#10280,#10277,#6579,.T.);
#12904=EDGE_CURVE('',#10280,#10275,#5477,.T.);
#12905=EDGE_CURVE('',#10281,#10282,#6580,.T.);
#12906=EDGE_CURVE('',#10283,#10281,#6581,.T.);
#12907=EDGE_CURVE('',#10283,#10284,#6582,.T.);
#12908=EDGE_CURVE('',#10284,#10282,#6583,.T.);
#12909=EDGE_CURVE('',#10282,#10285,#5478,.T.);
#12910=EDGE_CURVE('',#10285,#10284,#6584,.T.);
#12911=EDGE_CURVE('',#10285,#10286,#6585,.T.);
#12912=EDGE_CURVE('',#10286,#10283,#6586,.T.);
#12913=EDGE_CURVE('',#10286,#10281,#5479,.T.);
#12914=EDGE_CURVE('',#10287,#10288,#6587,.T.);
#12915=EDGE_CURVE('',#10289,#10287,#6588,.T.);
#12916=EDGE_CURVE('',#10289,#10290,#6589,.T.);
#12917=EDGE_CURVE('',#10290,#10288,#6590,.T.);
#12918=EDGE_CURVE('',#10288,#10291,#5480,.T.);
#12919=EDGE_CURVE('',#10291,#10290,#6591,.T.);
#12920=EDGE_CURVE('',#10291,#10292,#6592,.T.);
#12921=EDGE_CURVE('',#10292,#10289,#6593,.T.);
#12922=EDGE_CURVE('',#10292,#10287,#5481,.T.);
#12923=EDGE_CURVE('',#10293,#10294,#6594,.T.);
#12924=EDGE_CURVE('',#10295,#10293,#6595,.T.);
#12925=EDGE_CURVE('',#10295,#10296,#6596,.T.);
#12926=EDGE_CURVE('',#10296,#10294,#6597,.T.);
#12927=EDGE_CURVE('',#10294,#10297,#5482,.T.);
#12928=EDGE_CURVE('',#10297,#10296,#6598,.T.);
#12929=EDGE_CURVE('',#10297,#10298,#6599,.T.);
#12930=EDGE_CURVE('',#10298,#10295,#6600,.T.);
#12931=EDGE_CURVE('',#10298,#10293,#5483,.T.);
#12932=EDGE_CURVE('',#10299,#10300,#6601,.T.);
#12933=EDGE_CURVE('',#10301,#10299,#6602,.T.);
#12934=EDGE_CURVE('',#10301,#10302,#6603,.T.);
#12935=EDGE_CURVE('',#10302,#10300,#6604,.T.);
#12936=EDGE_CURVE('',#10300,#10303,#5484,.T.);
#12937=EDGE_CURVE('',#10303,#10302,#6605,.T.);
#12938=EDGE_CURVE('',#10303,#10304,#6606,.T.);
#12939=EDGE_CURVE('',#10304,#10301,#6607,.T.);
#12940=EDGE_CURVE('',#10304,#10299,#5485,.T.);
#12941=EDGE_CURVE('',#10305,#10306,#6608,.T.);
#12942=EDGE_CURVE('',#10307,#10305,#6609,.T.);
#12943=EDGE_CURVE('',#10307,#10308,#6610,.T.);
#12944=EDGE_CURVE('',#10308,#10306,#6611,.T.);
#12945=EDGE_CURVE('',#10306,#10309,#5486,.T.);
#12946=EDGE_CURVE('',#10309,#10308,#6612,.T.);
#12947=EDGE_CURVE('',#10309,#10310,#6613,.T.);
#12948=EDGE_CURVE('',#10310,#10307,#6614,.T.);
#12949=EDGE_CURVE('',#10310,#10305,#5487,.T.);
#12950=EDGE_CURVE('',#10311,#10312,#6615,.T.);
#12951=EDGE_CURVE('',#10313,#10311,#6616,.T.);
#12952=EDGE_CURVE('',#10313,#10314,#6617,.T.);
#12953=EDGE_CURVE('',#10314,#10312,#6618,.T.);
#12954=EDGE_CURVE('',#10312,#10315,#5488,.T.);
#12955=EDGE_CURVE('',#10315,#10314,#6619,.T.);
#12956=EDGE_CURVE('',#10315,#10316,#6620,.T.);
#12957=EDGE_CURVE('',#10316,#10313,#6621,.T.);
#12958=EDGE_CURVE('',#10316,#10311,#5489,.T.);
#12959=EDGE_CURVE('',#10317,#10318,#6622,.T.);
#12960=EDGE_CURVE('',#10319,#10317,#6623,.T.);
#12961=EDGE_CURVE('',#10319,#10320,#6624,.T.);
#12962=EDGE_CURVE('',#10320,#10318,#6625,.T.);
#12963=EDGE_CURVE('',#10318,#10321,#5490,.T.);
#12964=EDGE_CURVE('',#10321,#10320,#6626,.T.);
#12965=EDGE_CURVE('',#10321,#10322,#6627,.T.);
#12966=EDGE_CURVE('',#10322,#10319,#6628,.T.);
#12967=EDGE_CURVE('',#10322,#10317,#5491,.T.);
#12968=EDGE_CURVE('',#10323,#10323,#5492,.T.);
#12969=EDGE_CURVE('',#10323,#10324,#6629,.T.);
#12970=EDGE_CURVE('',#10324,#10324,#5493,.T.);
#12971=EDGE_CURVE('',#10325,#10325,#5494,.T.);
#12972=EDGE_CURVE('',#10325,#10326,#6630,.T.);
#12973=EDGE_CURVE('',#10326,#10326,#5495,.T.);
#12974=EDGE_CURVE('',#10327,#10327,#5496,.T.);
#12975=EDGE_CURVE('',#10328,#10328,#5497,.T.);
#12976=EDGE_CURVE('',#10328,#10327,#6631,.T.);
#12977=EDGE_CURVE('',#10212,#10328,#6632,.T.);
#12978=EDGE_CURVE('',#10329,#10329,#5498,.T.);
#12979=EDGE_CURVE('',#10330,#10330,#5499,.T.);
#12980=EDGE_CURVE('',#10330,#10265,#6633,.T.);
#12981=EDGE_CURVE('',#10268,#10329,#6634,.T.);
#12982=EDGE_CURVE('',#10331,#10331,#5500,.T.);
#12983=EDGE_CURVE('',#10332,#10332,#5501,.T.);
#12984=EDGE_CURVE('',#10332,#10331,#6635,.T.);
#17227=ORIENTED_EDGE('',*,*,#12791,.T.);
#17228=ORIENTED_EDGE('',*,*,#12792,.T.);
#17229=ORIENTED_EDGE('',*,*,#12793,.T.);
#17230=ORIENTED_EDGE('',*,*,#12794,.T.);
#17231=ORIENTED_EDGE('',*,*,#12795,.T.);
#17232=ORIENTED_EDGE('',*,*,#12793,.F.);
#17233=ORIENTED_EDGE('',*,*,#12794,.F.);
#17234=ORIENTED_EDGE('',*,*,#12795,.F.);
#17235=ORIENTED_EDGE('',*,*,#12796,.T.);
#17236=ORIENTED_EDGE('',*,*,#12797,.F.);
#17237=ORIENTED_EDGE('',*,*,#12798,.F.);
#17238=ORIENTED_EDGE('',*,*,#12796,.F.);
#17239=ORIENTED_EDGE('',*,*,#12799,.F.);
#17240=ORIENTED_EDGE('',*,*,#12800,.T.);
#17241=ORIENTED_EDGE('',*,*,#12791,.F.);
#17242=ORIENTED_EDGE('',*,*,#12792,.F.);
#17243=ORIENTED_EDGE('',*,*,#12800,.F.);
#17244=ORIENTED_EDGE('',*,*,#12797,.T.);
#17245=ORIENTED_EDGE('',*,*,#12798,.T.);
#17246=ORIENTED_EDGE('',*,*,#12801,.T.);
#17247=ORIENTED_EDGE('',*,*,#12802,.T.);
#17248=ORIENTED_EDGE('',*,*,#12801,.F.);
#17249=ORIENTED_EDGE('',*,*,#12802,.F.);
#17250=ORIENTED_EDGE('',*,*,#12803,.T.);
#17251=ORIENTED_EDGE('',*,*,#12804,.F.);
#17252=ORIENTED_EDGE('',*,*,#12805,.F.);
#17253=ORIENTED_EDGE('',*,*,#12806,.T.);
#17254=ORIENTED_EDGE('',*,*,#12807,.T.);
#17255=ORIENTED_EDGE('',*,*,#12808,.F.);
#17256=ORIENTED_EDGE('',*,*,#12807,.F.);
#17257=ORIENTED_EDGE('',*,*,#12809,.F.);
#17258=ORIENTED_EDGE('',*,*,#12810,.F.);
#17259=ORIENTED_EDGE('',*,*,#12809,.T.);
#17260=ORIENTED_EDGE('',*,*,#12806,.F.);
#17261=ORIENTED_EDGE('',*,*,#12811,.F.);
#17262=ORIENTED_EDGE('',*,*,#12812,.F.);
#17263=ORIENTED_EDGE('',*,*,#12811,.T.);
#17264=ORIENTED_EDGE('',*,*,#12805,.T.);
#17265=ORIENTED_EDGE('',*,*,#12813,.F.);
#17266=ORIENTED_EDGE('',*,*,#12814,.F.);
#17267=ORIENTED_EDGE('',*,*,#12815,.T.);
#17268=ORIENTED_EDGE('',*,*,#12816,.T.);
#17269=ORIENTED_EDGE('',*,*,#12817,.F.);
#17270=ORIENTED_EDGE('',*,*,#12816,.F.);
#17271=ORIENTED_EDGE('',*,*,#12818,.F.);
#17272=ORIENTED_EDGE('',*,*,#12819,.F.);
#17273=ORIENTED_EDGE('',*,*,#12818,.T.);
#17274=ORIENTED_EDGE('',*,*,#12815,.F.);
#17275=ORIENTED_EDGE('',*,*,#12820,.F.);
#17276=ORIENTED_EDGE('',*,*,#12821,.F.);
#17277=ORIENTED_EDGE('',*,*,#12820,.T.);
#17278=ORIENTED_EDGE('',*,*,#12814,.T.);
#17279=ORIENTED_EDGE('',*,*,#12822,.F.);
#17280=ORIENTED_EDGE('',*,*,#12823,.F.);
#17281=ORIENTED_EDGE('',*,*,#12824,.T.);
#17282=ORIENTED_EDGE('',*,*,#12825,.T.);
#17283=ORIENTED_EDGE('',*,*,#12826,.F.);
#17284=ORIENTED_EDGE('',*,*,#12825,.F.);
#17285=ORIENTED_EDGE('',*,*,#12827,.F.);
#17286=ORIENTED_EDGE('',*,*,#12828,.F.);
#17287=ORIENTED_EDGE('',*,*,#12827,.T.);
#17288=ORIENTED_EDGE('',*,*,#12824,.F.);
#17289=ORIENTED_EDGE('',*,*,#12829,.F.);
#17290=ORIENTED_EDGE('',*,*,#12830,.F.);
#17291=ORIENTED_EDGE('',*,*,#12829,.T.);
#17292=ORIENTED_EDGE('',*,*,#12823,.T.);
#17293=ORIENTED_EDGE('',*,*,#12831,.F.);
#17294=ORIENTED_EDGE('',*,*,#12832,.F.);
#17295=ORIENTED_EDGE('',*,*,#12833,.T.);
#17296=ORIENTED_EDGE('',*,*,#12834,.T.);
#17297=ORIENTED_EDGE('',*,*,#12835,.F.);
#17298=ORIENTED_EDGE('',*,*,#12834,.F.);
#17299=ORIENTED_EDGE('',*,*,#12836,.F.);
#17300=ORIENTED_EDGE('',*,*,#12837,.F.);
#17301=ORIENTED_EDGE('',*,*,#12836,.T.);
#17302=ORIENTED_EDGE('',*,*,#12833,.F.);
#17303=ORIENTED_EDGE('',*,*,#12838,.F.);
#17304=ORIENTED_EDGE('',*,*,#12839,.F.);
#17305=ORIENTED_EDGE('',*,*,#12838,.T.);
#17306=ORIENTED_EDGE('',*,*,#12832,.T.);
#17307=ORIENTED_EDGE('',*,*,#12840,.F.);
#17308=ORIENTED_EDGE('',*,*,#12841,.F.);
#17309=ORIENTED_EDGE('',*,*,#12842,.T.);
#17310=ORIENTED_EDGE('',*,*,#12843,.T.);
#17311=ORIENTED_EDGE('',*,*,#12844,.F.);
#17312=ORIENTED_EDGE('',*,*,#12843,.F.);
#17313=ORIENTED_EDGE('',*,*,#12845,.F.);
#17314=ORIENTED_EDGE('',*,*,#12846,.F.);
#17315=ORIENTED_EDGE('',*,*,#12845,.T.);
#17316=ORIENTED_EDGE('',*,*,#12842,.F.);
#17317=ORIENTED_EDGE('',*,*,#12847,.F.);
#17318=ORIENTED_EDGE('',*,*,#12848,.F.);
#17319=ORIENTED_EDGE('',*,*,#12847,.T.);
#17320=ORIENTED_EDGE('',*,*,#12841,.T.);
#17321=ORIENTED_EDGE('',*,*,#12849,.F.);
#17322=ORIENTED_EDGE('',*,*,#12850,.F.);
#17323=ORIENTED_EDGE('',*,*,#12851,.T.);
#17324=ORIENTED_EDGE('',*,*,#12852,.T.);
#17325=ORIENTED_EDGE('',*,*,#12853,.F.);
#17326=ORIENTED_EDGE('',*,*,#12852,.F.);
#17327=ORIENTED_EDGE('',*,*,#12854,.F.);
#17328=ORIENTED_EDGE('',*,*,#12855,.F.);
#17329=ORIENTED_EDGE('',*,*,#12854,.T.);
#17330=ORIENTED_EDGE('',*,*,#12851,.F.);
#17331=ORIENTED_EDGE('',*,*,#12856,.F.);
#17332=ORIENTED_EDGE('',*,*,#12857,.F.);
#17333=ORIENTED_EDGE('',*,*,#12856,.T.);
#17334=ORIENTED_EDGE('',*,*,#12850,.T.);
#17335=ORIENTED_EDGE('',*,*,#12858,.F.);
#17336=ORIENTED_EDGE('',*,*,#12859,.F.);
#17337=ORIENTED_EDGE('',*,*,#12860,.T.);
#17338=ORIENTED_EDGE('',*,*,#12861,.T.);
#17339=ORIENTED_EDGE('',*,*,#12862,.F.);
#17340=ORIENTED_EDGE('',*,*,#12861,.F.);
#17341=ORIENTED_EDGE('',*,*,#12863,.F.);
#17342=ORIENTED_EDGE('',*,*,#12864,.F.);
#17343=ORIENTED_EDGE('',*,*,#12863,.T.);
#17344=ORIENTED_EDGE('',*,*,#12860,.F.);
#17345=ORIENTED_EDGE('',*,*,#12865,.F.);
#17346=ORIENTED_EDGE('',*,*,#12866,.F.);
#17347=ORIENTED_EDGE('',*,*,#12865,.T.);
#17348=ORIENTED_EDGE('',*,*,#12859,.T.);
#17349=ORIENTED_EDGE('',*,*,#12867,.F.);
#17350=ORIENTED_EDGE('',*,*,#12868,.F.);
#17351=ORIENTED_EDGE('',*,*,#12869,.T.);
#17352=ORIENTED_EDGE('',*,*,#12870,.T.);
#17353=ORIENTED_EDGE('',*,*,#12871,.F.);
#17354=ORIENTED_EDGE('',*,*,#12870,.F.);
#17355=ORIENTED_EDGE('',*,*,#12872,.F.);
#17356=ORIENTED_EDGE('',*,*,#12873,.F.);
#17357=ORIENTED_EDGE('',*,*,#12872,.T.);
#17358=ORIENTED_EDGE('',*,*,#12869,.F.);
#17359=ORIENTED_EDGE('',*,*,#12874,.F.);
#17360=ORIENTED_EDGE('',*,*,#12875,.F.);
#17361=ORIENTED_EDGE('',*,*,#12874,.T.);
#17362=ORIENTED_EDGE('',*,*,#12868,.T.);
#17363=ORIENTED_EDGE('',*,*,#12876,.F.);
#17364=ORIENTED_EDGE('',*,*,#12877,.F.);
#17365=ORIENTED_EDGE('',*,*,#12878,.T.);
#17366=ORIENTED_EDGE('',*,*,#12879,.T.);
#17367=ORIENTED_EDGE('',*,*,#12880,.F.);
#17368=ORIENTED_EDGE('',*,*,#12879,.F.);
#17369=ORIENTED_EDGE('',*,*,#12881,.F.);
#17370=ORIENTED_EDGE('',*,*,#12882,.F.);
#17371=ORIENTED_EDGE('',*,*,#12883,.F.);
#17372=ORIENTED_EDGE('',*,*,#12881,.T.);
#17373=ORIENTED_EDGE('',*,*,#12878,.F.);
#17374=ORIENTED_EDGE('',*,*,#12884,.F.);
#17375=ORIENTED_EDGE('',*,*,#12885,.F.);
#17376=ORIENTED_EDGE('',*,*,#12884,.T.);
#17377=ORIENTED_EDGE('',*,*,#12877,.T.);
#17378=ORIENTED_EDGE('',*,*,#12886,.F.);
#17379=ORIENTED_EDGE('',*,*,#12887,.F.);
#17380=ORIENTED_EDGE('',*,*,#12888,.F.);
#17381=ORIENTED_EDGE('',*,*,#12889,.T.);
#17382=ORIENTED_EDGE('',*,*,#12890,.T.);
#17383=ORIENTED_EDGE('',*,*,#12891,.F.);
#17384=ORIENTED_EDGE('',*,*,#12890,.F.);
#17385=ORIENTED_EDGE('',*,*,#12892,.F.);
#17386=ORIENTED_EDGE('',*,*,#12893,.F.);
#17387=ORIENTED_EDGE('',*,*,#12892,.T.);
#17388=ORIENTED_EDGE('',*,*,#12889,.F.);
#17389=ORIENTED_EDGE('',*,*,#12894,.F.);
#17390=ORIENTED_EDGE('',*,*,#12895,.F.);
#17391=ORIENTED_EDGE('',*,*,#12894,.T.);
#17392=ORIENTED_EDGE('',*,*,#12888,.T.);
#17393=ORIENTED_EDGE('',*,*,#12896,.F.);
#17394=ORIENTED_EDGE('',*,*,#12897,.F.);
#17395=ORIENTED_EDGE('',*,*,#12898,.T.);
#17396=ORIENTED_EDGE('',*,*,#12899,.T.);
#17397=ORIENTED_EDGE('',*,*,#12900,.F.);
#17398=ORIENTED_EDGE('',*,*,#12899,.F.);
#17399=ORIENTED_EDGE('',*,*,#12901,.F.);
#17400=ORIENTED_EDGE('',*,*,#12902,.F.);
#17401=ORIENTED_EDGE('',*,*,#12901,.T.);
#17402=ORIENTED_EDGE('',*,*,#12898,.F.);
#17403=ORIENTED_EDGE('',*,*,#12903,.F.);
#17404=ORIENTED_EDGE('',*,*,#12904,.F.);
#17405=ORIENTED_EDGE('',*,*,#12903,.T.);
#17406=ORIENTED_EDGE('',*,*,#12897,.T.);
#17407=ORIENTED_EDGE('',*,*,#12905,.F.);
#17408=ORIENTED_EDGE('',*,*,#12906,.F.);
#17409=ORIENTED_EDGE('',*,*,#12907,.T.);
#17410=ORIENTED_EDGE('',*,*,#12908,.T.);
#17411=ORIENTED_EDGE('',*,*,#12909,.F.);
#17412=ORIENTED_EDGE('',*,*,#12908,.F.);
#17413=ORIENTED_EDGE('',*,*,#12910,.F.);
#17414=ORIENTED_EDGE('',*,*,#12911,.F.);
#17415=ORIENTED_EDGE('',*,*,#12910,.T.);
#17416=ORIENTED_EDGE('',*,*,#12907,.F.);
#17417=ORIENTED_EDGE('',*,*,#12912,.F.);
#17418=ORIENTED_EDGE('',*,*,#12913,.F.);
#17419=ORIENTED_EDGE('',*,*,#12912,.T.);
#17420=ORIENTED_EDGE('',*,*,#12906,.T.);
#17421=ORIENTED_EDGE('',*,*,#12914,.F.);
#17422=ORIENTED_EDGE('',*,*,#12915,.F.);
#17423=ORIENTED_EDGE('',*,*,#12916,.T.);
#17424=ORIENTED_EDGE('',*,*,#12917,.T.);
#17425=ORIENTED_EDGE('',*,*,#12918,.F.);
#17426=ORIENTED_EDGE('',*,*,#12917,.F.);
#17427=ORIENTED_EDGE('',*,*,#12919,.F.);
#17428=ORIENTED_EDGE('',*,*,#12920,.F.);
#17429=ORIENTED_EDGE('',*,*,#12919,.T.);
#17430=ORIENTED_EDGE('',*,*,#12916,.F.);
#17431=ORIENTED_EDGE('',*,*,#12921,.F.);
#17432=ORIENTED_EDGE('',*,*,#12922,.F.);
#17433=ORIENTED_EDGE('',*,*,#12921,.T.);
#17434=ORIENTED_EDGE('',*,*,#12915,.T.);
#17435=ORIENTED_EDGE('',*,*,#12923,.F.);
#17436=ORIENTED_EDGE('',*,*,#12924,.F.);
#17437=ORIENTED_EDGE('',*,*,#12925,.T.);
#17438=ORIENTED_EDGE('',*,*,#12926,.T.);
#17439=ORIENTED_EDGE('',*,*,#12927,.F.);
#17440=ORIENTED_EDGE('',*,*,#12926,.F.);
#17441=ORIENTED_EDGE('',*,*,#12928,.F.);
#17442=ORIENTED_EDGE('',*,*,#12929,.F.);
#17443=ORIENTED_EDGE('',*,*,#12928,.T.);
#17444=ORIENTED_EDGE('',*,*,#12925,.F.);
#17445=ORIENTED_EDGE('',*,*,#12930,.F.);
#17446=ORIENTED_EDGE('',*,*,#12931,.F.);
#17447=ORIENTED_EDGE('',*,*,#12930,.T.);
#17448=ORIENTED_EDGE('',*,*,#12924,.T.);
#17449=ORIENTED_EDGE('',*,*,#12932,.F.);
#17450=ORIENTED_EDGE('',*,*,#12933,.F.);
#17451=ORIENTED_EDGE('',*,*,#12934,.T.);
#17452=ORIENTED_EDGE('',*,*,#12935,.T.);
#17453=ORIENTED_EDGE('',*,*,#12936,.F.);
#17454=ORIENTED_EDGE('',*,*,#12935,.F.);
#17455=ORIENTED_EDGE('',*,*,#12937,.F.);
#17456=ORIENTED_EDGE('',*,*,#12938,.F.);
#17457=ORIENTED_EDGE('',*,*,#12937,.T.);
#17458=ORIENTED_EDGE('',*,*,#12934,.F.);
#17459=ORIENTED_EDGE('',*,*,#12939,.F.);
#17460=ORIENTED_EDGE('',*,*,#12940,.F.);
#17461=ORIENTED_EDGE('',*,*,#12939,.T.);
#17462=ORIENTED_EDGE('',*,*,#12933,.T.);
#17463=ORIENTED_EDGE('',*,*,#12941,.F.);
#17464=ORIENTED_EDGE('',*,*,#12942,.F.);
#17465=ORIENTED_EDGE('',*,*,#12943,.T.);
#17466=ORIENTED_EDGE('',*,*,#12944,.T.);
#17467=ORIENTED_EDGE('',*,*,#12945,.F.);
#17468=ORIENTED_EDGE('',*,*,#12944,.F.);
#17469=ORIENTED_EDGE('',*,*,#12946,.F.);
#17470=ORIENTED_EDGE('',*,*,#12947,.F.);
#17471=ORIENTED_EDGE('',*,*,#12946,.T.);
#17472=ORIENTED_EDGE('',*,*,#12943,.F.);
#17473=ORIENTED_EDGE('',*,*,#12948,.F.);
#17474=ORIENTED_EDGE('',*,*,#12949,.F.);
#17475=ORIENTED_EDGE('',*,*,#12948,.T.);
#17476=ORIENTED_EDGE('',*,*,#12942,.T.);
#17477=ORIENTED_EDGE('',*,*,#12950,.F.);
#17478=ORIENTED_EDGE('',*,*,#12951,.F.);
#17479=ORIENTED_EDGE('',*,*,#12952,.T.);
#17480=ORIENTED_EDGE('',*,*,#12953,.T.);
#17481=ORIENTED_EDGE('',*,*,#12954,.F.);
#17482=ORIENTED_EDGE('',*,*,#12953,.F.);
#17483=ORIENTED_EDGE('',*,*,#12955,.F.);
#17484=ORIENTED_EDGE('',*,*,#12956,.F.);
#17485=ORIENTED_EDGE('',*,*,#12955,.T.);
#17486=ORIENTED_EDGE('',*,*,#12952,.F.);
#17487=ORIENTED_EDGE('',*,*,#12957,.F.);
#17488=ORIENTED_EDGE('',*,*,#12958,.F.);
#17489=ORIENTED_EDGE('',*,*,#12957,.T.);
#17490=ORIENTED_EDGE('',*,*,#12951,.T.);
#17491=ORIENTED_EDGE('',*,*,#12959,.F.);
#17492=ORIENTED_EDGE('',*,*,#12960,.F.);
#17493=ORIENTED_EDGE('',*,*,#12961,.T.);
#17494=ORIENTED_EDGE('',*,*,#12962,.T.);
#17495=ORIENTED_EDGE('',*,*,#12963,.F.);
#17496=ORIENTED_EDGE('',*,*,#12962,.F.);
#17497=ORIENTED_EDGE('',*,*,#12964,.F.);
#17498=ORIENTED_EDGE('',*,*,#12965,.F.);
#17499=ORIENTED_EDGE('',*,*,#12964,.T.);
#17500=ORIENTED_EDGE('',*,*,#12961,.F.);
#17501=ORIENTED_EDGE('',*,*,#12966,.F.);
#17502=ORIENTED_EDGE('',*,*,#12967,.F.);
#17503=ORIENTED_EDGE('',*,*,#12966,.T.);
#17504=ORIENTED_EDGE('',*,*,#12960,.T.);
#17505=ORIENTED_EDGE('',*,*,#12968,.F.);
#17506=ORIENTED_EDGE('',*,*,#12969,.T.);
#17507=ORIENTED_EDGE('',*,*,#12970,.F.);
#17508=ORIENTED_EDGE('',*,*,#12969,.F.);
#17509=ORIENTED_EDGE('',*,*,#12971,.F.);
#17510=ORIENTED_EDGE('',*,*,#12972,.T.);
#17511=ORIENTED_EDGE('',*,*,#12973,.T.);
#17512=ORIENTED_EDGE('',*,*,#12972,.F.);
#17513=ORIENTED_EDGE('',*,*,#12973,.F.);
#17514=ORIENTED_EDGE('',*,*,#12970,.T.);
#17515=ORIENTED_EDGE('',*,*,#12974,.F.);
#17516=ORIENTED_EDGE('',*,*,#12971,.T.);
#17517=ORIENTED_EDGE('',*,*,#12968,.T.);
#17518=ORIENTED_EDGE('',*,*,#12975,.F.);
#17519=ORIENTED_EDGE('',*,*,#12976,.T.);
#17520=ORIENTED_EDGE('',*,*,#12974,.T.);
#17521=ORIENTED_EDGE('',*,*,#12976,.F.);
#17522=ORIENTED_EDGE('',*,*,#12803,.F.);
#17523=ORIENTED_EDGE('',*,*,#12977,.T.);
#17524=ORIENTED_EDGE('',*,*,#12975,.T.);
#17525=ORIENTED_EDGE('',*,*,#12977,.F.);
#17526=ORIENTED_EDGE('',*,*,#12799,.T.);
#17527=ORIENTED_EDGE('',*,*,#12978,.F.);
#17528=ORIENTED_EDGE('',*,*,#12979,.F.);
#17529=ORIENTED_EDGE('',*,*,#12980,.T.);
#17530=ORIENTED_EDGE('',*,*,#12882,.T.);
#17531=ORIENTED_EDGE('',*,*,#12883,.T.);
#17532=ORIENTED_EDGE('',*,*,#12885,.T.);
#17533=ORIENTED_EDGE('',*,*,#12981,.T.);
#17534=ORIENTED_EDGE('',*,*,#12978,.T.);
#17535=ORIENTED_EDGE('',*,*,#12981,.F.);
#17536=ORIENTED_EDGE('',*,*,#12886,.T.);
#17537=ORIENTED_EDGE('',*,*,#12876,.T.);
#17538=ORIENTED_EDGE('',*,*,#12880,.T.);
#17539=ORIENTED_EDGE('',*,*,#12980,.F.);
#17540=ORIENTED_EDGE('',*,*,#12810,.T.);
#17541=ORIENTED_EDGE('',*,*,#12812,.T.);
#17542=ORIENTED_EDGE('',*,*,#12804,.T.);
#17543=ORIENTED_EDGE('',*,*,#12808,.T.);
#17544=ORIENTED_EDGE('',*,*,#12819,.T.);
#17545=ORIENTED_EDGE('',*,*,#12821,.T.);
#17546=ORIENTED_EDGE('',*,*,#12813,.T.);
#17547=ORIENTED_EDGE('',*,*,#12817,.T.);
#17548=ORIENTED_EDGE('',*,*,#12828,.T.);
#17549=ORIENTED_EDGE('',*,*,#12830,.T.);
#17550=ORIENTED_EDGE('',*,*,#12822,.T.);
#17551=ORIENTED_EDGE('',*,*,#12826,.T.);
#17552=ORIENTED_EDGE('',*,*,#12837,.T.);
#17553=ORIENTED_EDGE('',*,*,#12839,.T.);
#17554=ORIENTED_EDGE('',*,*,#12831,.T.);
#17555=ORIENTED_EDGE('',*,*,#12835,.T.);
#17556=ORIENTED_EDGE('',*,*,#12846,.T.);
#17557=ORIENTED_EDGE('',*,*,#12848,.T.);
#17558=ORIENTED_EDGE('',*,*,#12840,.T.);
#17559=ORIENTED_EDGE('',*,*,#12844,.T.);
#17560=ORIENTED_EDGE('',*,*,#12855,.T.);
#17561=ORIENTED_EDGE('',*,*,#12857,.T.);
#17562=ORIENTED_EDGE('',*,*,#12849,.T.);
#17563=ORIENTED_EDGE('',*,*,#12853,.T.);
#17564=ORIENTED_EDGE('',*,*,#12864,.T.);
#17565=ORIENTED_EDGE('',*,*,#12866,.T.);
#17566=ORIENTED_EDGE('',*,*,#12858,.T.);
#17567=ORIENTED_EDGE('',*,*,#12862,.T.);
#17568=ORIENTED_EDGE('',*,*,#12873,.T.);
#17569=ORIENTED_EDGE('',*,*,#12875,.T.);
#17570=ORIENTED_EDGE('',*,*,#12867,.T.);
#17571=ORIENTED_EDGE('',*,*,#12871,.T.);
#17572=ORIENTED_EDGE('',*,*,#12893,.T.);
#17573=ORIENTED_EDGE('',*,*,#12895,.T.);
#17574=ORIENTED_EDGE('',*,*,#12887,.T.);
#17575=ORIENTED_EDGE('',*,*,#12891,.T.);
#17576=ORIENTED_EDGE('',*,*,#12902,.T.);
#17577=ORIENTED_EDGE('',*,*,#12904,.T.);
#17578=ORIENTED_EDGE('',*,*,#12896,.T.);
#17579=ORIENTED_EDGE('',*,*,#12900,.T.);
#17580=ORIENTED_EDGE('',*,*,#12911,.T.);
#17581=ORIENTED_EDGE('',*,*,#12913,.T.);
#17582=ORIENTED_EDGE('',*,*,#12905,.T.);
#17583=ORIENTED_EDGE('',*,*,#12909,.T.);
#17584=ORIENTED_EDGE('',*,*,#12920,.T.);
#17585=ORIENTED_EDGE('',*,*,#12922,.T.);
#17586=ORIENTED_EDGE('',*,*,#12914,.T.);
#17587=ORIENTED_EDGE('',*,*,#12918,.T.);
#17588=ORIENTED_EDGE('',*,*,#12929,.T.);
#17589=ORIENTED_EDGE('',*,*,#12931,.T.);
#17590=ORIENTED_EDGE('',*,*,#12923,.T.);
#17591=ORIENTED_EDGE('',*,*,#12927,.T.);
#17592=ORIENTED_EDGE('',*,*,#12938,.T.);
#17593=ORIENTED_EDGE('',*,*,#12940,.T.);
#17594=ORIENTED_EDGE('',*,*,#12932,.T.);
#17595=ORIENTED_EDGE('',*,*,#12936,.T.);
#17596=ORIENTED_EDGE('',*,*,#12947,.T.);
#17597=ORIENTED_EDGE('',*,*,#12949,.T.);
#17598=ORIENTED_EDGE('',*,*,#12941,.T.);
#17599=ORIENTED_EDGE('',*,*,#12945,.T.);
#17600=ORIENTED_EDGE('',*,*,#12956,.T.);
#17601=ORIENTED_EDGE('',*,*,#12958,.T.);
#17602=ORIENTED_EDGE('',*,*,#12950,.T.);
#17603=ORIENTED_EDGE('',*,*,#12954,.T.);
#17604=ORIENTED_EDGE('',*,*,#12965,.T.);
#17605=ORIENTED_EDGE('',*,*,#12967,.T.);
#17606=ORIENTED_EDGE('',*,*,#12959,.T.);
#17607=ORIENTED_EDGE('',*,*,#12963,.T.);
#17608=ORIENTED_EDGE('',*,*,#12979,.T.);
#17609=ORIENTED_EDGE('',*,*,#12982,.F.);
#17610=ORIENTED_EDGE('',*,*,#12983,.F.);
#17611=ORIENTED_EDGE('',*,*,#12984,.T.);
#17612=ORIENTED_EDGE('',*,*,#12982,.T.);
#17613=ORIENTED_EDGE('',*,*,#12984,.F.);
#17614=ORIENTED_EDGE('',*,*,#12983,.T.);
#21943=CONICAL_SURFACE('',#24375,0.589393398282202,0.392699081698718);
#21944=CONICAL_SURFACE('',#24383,0.58,0.785398163397448);
#21945=CONICAL_SURFACE('',#24385,0.585,0.785398163397445);
#21946=CONICAL_SURFACE('',#24509,0.39,0.785398163397449);
#22464=ADVANCED_FACE('',(#2725),#21943,.T.);
#22465=ADVANCED_FACE('',(#2726),#1038,.T.);
#22466=ADVANCED_FACE('',(#2727),#21944,.T.);
#22467=ADVANCED_FACE('',(#2728),#21945,.T.);
#22468=ADVANCED_FACE('',(#2729,#1388),#1676,.T.);
#22469=ADVANCED_FACE('',(#2730),#1677,.F.);
#22470=ADVANCED_FACE('',(#2731),#1678,.F.);
#22471=ADVANCED_FACE('',(#2732),#1679,.F.);
#22472=ADVANCED_FACE('',(#2733),#1680,.T.);
#22473=ADVANCED_FACE('',(#2734),#1681,.F.);
#22474=ADVANCED_FACE('',(#2735),#1682,.F.);
#22475=ADVANCED_FACE('',(#2736),#1683,.F.);
#22476=ADVANCED_FACE('',(#2737),#1684,.T.);
#22477=ADVANCED_FACE('',(#2738),#1685,.F.);
#22478=ADVANCED_FACE('',(#2739),#1686,.F.);
#22479=ADVANCED_FACE('',(#2740),#1687,.F.);
#22480=ADVANCED_FACE('',(#2741),#1688,.T.);
#22481=ADVANCED_FACE('',(#2742),#1689,.F.);
#22482=ADVANCED_FACE('',(#2743),#1690,.F.);
#22483=ADVANCED_FACE('',(#2744),#1691,.F.);
#22484=ADVANCED_FACE('',(#2745),#1692,.T.);
#22485=ADVANCED_FACE('',(#2746),#1693,.F.);
#22486=ADVANCED_FACE('',(#2747),#1694,.F.);
#22487=ADVANCED_FACE('',(#2748),#1695,.F.);
#22488=ADVANCED_FACE('',(#2749),#1696,.T.);
#22489=ADVANCED_FACE('',(#2750),#1697,.F.);
#22490=ADVANCED_FACE('',(#2751),#1698,.F.);
#22491=ADVANCED_FACE('',(#2752),#1699,.F.);
#22492=ADVANCED_FACE('',(#2753),#1700,.T.);
#22493=ADVANCED_FACE('',(#2754),#1701,.F.);
#22494=ADVANCED_FACE('',(#2755),#1702,.F.);
#22495=ADVANCED_FACE('',(#2756),#1703,.F.);
#22496=ADVANCED_FACE('',(#2757),#1704,.T.);
#22497=ADVANCED_FACE('',(#2758),#1705,.F.);
#22498=ADVANCED_FACE('',(#2759),#1706,.F.);
#22499=ADVANCED_FACE('',(#2760),#1707,.F.);
#22500=ADVANCED_FACE('',(#2761),#1708,.T.);
#22501=ADVANCED_FACE('',(#2762),#1709,.F.);
#22502=ADVANCED_FACE('',(#2763),#1710,.F.);
#22503=ADVANCED_FACE('',(#2764),#1711,.F.);
#22504=ADVANCED_FACE('',(#2765),#1712,.T.);
#22505=ADVANCED_FACE('',(#2766),#1713,.F.);
#22506=ADVANCED_FACE('',(#2767),#1714,.F.);
#22507=ADVANCED_FACE('',(#2768),#1715,.F.);
#22508=ADVANCED_FACE('',(#2769),#1716,.T.);
#22509=ADVANCED_FACE('',(#2770),#1717,.F.);
#22510=ADVANCED_FACE('',(#2771),#1718,.F.);
#22511=ADVANCED_FACE('',(#2772),#1719,.F.);
#22512=ADVANCED_FACE('',(#2773),#1720,.T.);
#22513=ADVANCED_FACE('',(#2774),#1721,.F.);
#22514=ADVANCED_FACE('',(#2775),#1722,.F.);
#22515=ADVANCED_FACE('',(#2776),#1723,.F.);
#22516=ADVANCED_FACE('',(#2777),#1724,.T.);
#22517=ADVANCED_FACE('',(#2778),#1725,.F.);
#22518=ADVANCED_FACE('',(#2779),#1726,.F.);
#22519=ADVANCED_FACE('',(#2780),#1727,.F.);
#22520=ADVANCED_FACE('',(#2781),#1728,.T.);
#22521=ADVANCED_FACE('',(#2782),#1729,.F.);
#22522=ADVANCED_FACE('',(#2783),#1730,.F.);
#22523=ADVANCED_FACE('',(#2784),#1731,.F.);
#22524=ADVANCED_FACE('',(#2785),#1732,.T.);
#22525=ADVANCED_FACE('',(#2786),#1733,.F.);
#22526=ADVANCED_FACE('',(#2787),#1734,.F.);
#22527=ADVANCED_FACE('',(#2788),#1735,.F.);
#22528=ADVANCED_FACE('',(#2789),#1736,.T.);
#22529=ADVANCED_FACE('',(#2790),#1737,.F.);
#22530=ADVANCED_FACE('',(#2791),#1738,.F.);
#22531=ADVANCED_FACE('',(#2792),#1739,.F.);
#22532=ADVANCED_FACE('',(#2793),#1740,.T.);
#22533=ADVANCED_FACE('',(#2794),#1741,.F.);
#22534=ADVANCED_FACE('',(#2795),#1742,.F.);
#22535=ADVANCED_FACE('',(#2796),#1743,.F.);
#22536=ADVANCED_FACE('',(#2797),#1744,.T.);
#22537=ADVANCED_FACE('',(#2798),#1745,.F.);
#22538=ADVANCED_FACE('',(#2799),#1746,.F.);
#22539=ADVANCED_FACE('',(#2800),#1747,.F.);
#22540=ADVANCED_FACE('',(#2801),#1748,.T.);
#22541=ADVANCED_FACE('',(#2802),#1039,.T.);
#22542=ADVANCED_FACE('',(#2803),#1040,.F.);
#22543=ADVANCED_FACE('',(#2804,#1389),#1749,.F.);
#22544=ADVANCED_FACE('',(#2805,#1390),#1750,.T.);
#22545=ADVANCED_FACE('',(#2806),#1751,.T.);
#22546=ADVANCED_FACE('',(#2807),#21946,.T.);
#22547=ADVANCED_FACE('',(#2808),#1041,.T.);
#22548=ADVANCED_FACE('',(#2809,#1391),#1752,.T.);
#22549=ADVANCED_FACE('',(#2810,#1392,#1393,#1394,#1395,#1396,#1397,#1398,
#1399,#1400,#1401,#1402,#1403,#1404,#1405,#1406,#1407,#1408),#1042,.T.);
#22550=ADVANCED_FACE('',(#2811,#1409),#1753,.T.);
#22551=ADVANCED_FACE('',(#2812),#1043,.T.);
#22552=ADVANCED_FACE('',(#2813),#1754,.T.);
#23311=CLOSED_SHELL('',(#22464,#22465,#22466,#22467,#22468,#22469,#22470,
#22471,#22472,#22473,#22474,#22475,#22476,#22477,#22478,#22479,#22480,#22481,
#22482,#22483,#22484,#22485,#22486,#22487,#22488,#22489,#22490,#22491,#22492,
#22493,#22494,#22495,#22496,#22497,#22498,#22499,#22500,#22501,#22502,#22503,
#22504,#22505,#22506,#22507,#22508,#22509,#22510,#22511,#22512,#22513,#22514,
#22515,#22516,#22517,#22518,#22519,#22520,#22521,#22522,#22523,#22524,#22525,
#22526,#22527,#22528,#22529,#22530,#22531,#22532,#22533,#22534,#22535,#22536,
#22537,#22538,#22539,#22540,#22541,#22542,#22543,#22544,#22545,#22546,#22547,
#22548,#22549,#22550,#22551,#22552));
#24374=AXIS2_PLACEMENT_3D('',#35554,#28057,#28058);
#24375=AXIS2_PLACEMENT_3D('',#35555,#28059,#28060);
#24376=AXIS2_PLACEMENT_3D('',#35558,#28061,#28062);
#24377=AXIS2_PLACEMENT_3D('',#35559,#28063,#28064);
#24378=AXIS2_PLACEMENT_3D('',#35563,#28066,#28067);
#24379=AXIS2_PLACEMENT_3D('',#35564,#28068,#28069);
#24380=AXIS2_PLACEMENT_3D('',#35565,#28070,#28071);
#24381=AXIS2_PLACEMENT_3D('',#35569,#28073,#28074);
#24382=AXIS2_PLACEMENT_3D('',#35570,#28075,#28076);
#24383=AXIS2_PLACEMENT_3D('',#35571,#28077,#28078);
#24384=AXIS2_PLACEMENT_3D('',#35573,#28079,#28080);
#24385=AXIS2_PLACEMENT_3D('',#35575,#28082,#28083);
#24386=AXIS2_PLACEMENT_3D('',#35578,#28085,#28086);
#24387=AXIS2_PLACEMENT_3D('',#35579,#28087,#28088);
#24388=AXIS2_PLACEMENT_3D('',#35581,#28089,#28090);
#24389=AXIS2_PLACEMENT_3D('',#35582,#28091,#28092);
#24390=AXIS2_PLACEMENT_3D('',#35591,#28097,#28098);
#24391=AXIS2_PLACEMENT_3D('',#35593,#28099,#28100);
#24392=AXIS2_PLACEMENT_3D('',#35595,#28102,#28103);
#24393=AXIS2_PLACEMENT_3D('',#35599,#28106,#28107);
#24394=AXIS2_PLACEMENT_3D('',#35600,#28108,#28109);
#24395=AXIS2_PLACEMENT_3D('',#35601,#28110,#28111);
#24396=AXIS2_PLACEMENT_3D('',#35610,#28116,#28117);
#24397=AXIS2_PLACEMENT_3D('',#35612,#28118,#28119);
#24398=AXIS2_PLACEMENT_3D('',#35614,#28121,#28122);
#24399=AXIS2_PLACEMENT_3D('',#35618,#28125,#28126);
#24400=AXIS2_PLACEMENT_3D('',#35619,#28127,#28128);
#24401=AXIS2_PLACEMENT_3D('',#35620,#28129,#28130);
#24402=AXIS2_PLACEMENT_3D('',#35629,#28135,#28136);
#24403=AXIS2_PLACEMENT_3D('',#35631,#28137,#28138);
#24404=AXIS2_PLACEMENT_3D('',#35633,#28140,#28141);
#24405=AXIS2_PLACEMENT_3D('',#35637,#28144,#28145);
#24406=AXIS2_PLACEMENT_3D('',#35638,#28146,#28147);
#24407=AXIS2_PLACEMENT_3D('',#35639,#28148,#28149);
#24408=AXIS2_PLACEMENT_3D('',#35648,#28154,#28155);
#24409=AXIS2_PLACEMENT_3D('',#35650,#28156,#28157);
#24410=AXIS2_PLACEMENT_3D('',#35652,#28159,#28160);
#24411=AXIS2_PLACEMENT_3D('',#35656,#28163,#28164);
#24412=AXIS2_PLACEMENT_3D('',#35657,#28165,#28166);
#24413=AXIS2_PLACEMENT_3D('',#35658,#28167,#28168);
#24414=AXIS2_PLACEMENT_3D('',#35667,#28173,#28174);
#24415=AXIS2_PLACEMENT_3D('',#35669,#28175,#28176);
#24416=AXIS2_PLACEMENT_3D('',#35671,#28178,#28179);
#24417=AXIS2_PLACEMENT_3D('',#35675,#28182,#28183);
#24418=AXIS2_PLACEMENT_3D('',#35676,#28184,#28185);
#24419=AXIS2_PLACEMENT_3D('',#35677,#28186,#28187);
#24420=AXIS2_PLACEMENT_3D('',#35686,#28192,#28193);
#24421=AXIS2_PLACEMENT_3D('',#35688,#28194,#28195);
#24422=AXIS2_PLACEMENT_3D('',#35690,#28197,#28198);
#24423=AXIS2_PLACEMENT_3D('',#35694,#28201,#28202);
#24424=AXIS2_PLACEMENT_3D('',#35695,#28203,#28204);
#24425=AXIS2_PLACEMENT_3D('',#35696,#28205,#28206);
#24426=AXIS2_PLACEMENT_3D('',#35705,#28211,#28212);
#24427=AXIS2_PLACEMENT_3D('',#35707,#28213,#28214);
#24428=AXIS2_PLACEMENT_3D('',#35709,#28216,#28217);
#24429=AXIS2_PLACEMENT_3D('',#35713,#28220,#28221);
#24430=AXIS2_PLACEMENT_3D('',#35714,#28222,#28223);
#24431=AXIS2_PLACEMENT_3D('',#35715,#28224,#28225);
#24432=AXIS2_PLACEMENT_3D('',#35724,#28230,#28231);
#24433=AXIS2_PLACEMENT_3D('',#35726,#28232,#28233);
#24434=AXIS2_PLACEMENT_3D('',#35728,#28235,#28236);
#24435=AXIS2_PLACEMENT_3D('',#35732,#28239,#28240);
#24436=AXIS2_PLACEMENT_3D('',#35733,#28241,#28242);
#24437=AXIS2_PLACEMENT_3D('',#35734,#28243,#28244);
#24438=AXIS2_PLACEMENT_3D('',#35743,#28249,#28250);
#24439=AXIS2_PLACEMENT_3D('',#35745,#28251,#28252);
#24440=AXIS2_PLACEMENT_3D('',#35748,#28254,#28255);
#24441=AXIS2_PLACEMENT_3D('',#35749,#28256,#28257);
#24442=AXIS2_PLACEMENT_3D('',#35753,#28260,#28261);
#24443=AXIS2_PLACEMENT_3D('',#35755,#28262,#28263);
#24444=AXIS2_PLACEMENT_3D('',#35756,#28264,#28265);
#24445=AXIS2_PLACEMENT_3D('',#35757,#28266,#28267);
#24446=AXIS2_PLACEMENT_3D('',#35766,#28272,#28273);
#24447=AXIS2_PLACEMENT_3D('',#35768,#28274,#28275);
#24448=AXIS2_PLACEMENT_3D('',#35770,#28277,#28278);
#24449=AXIS2_PLACEMENT_3D('',#35774,#28281,#28282);
#24450=AXIS2_PLACEMENT_3D('',#35775,#28283,#28284);
#24451=AXIS2_PLACEMENT_3D('',#35776,#28285,#28286);
#24452=AXIS2_PLACEMENT_3D('',#35785,#28291,#28292);
#24453=AXIS2_PLACEMENT_3D('',#35787,#28293,#28294);
#24454=AXIS2_PLACEMENT_3D('',#35789,#28296,#28297);
#24455=AXIS2_PLACEMENT_3D('',#35793,#28300,#28301);
#24456=AXIS2_PLACEMENT_3D('',#35794,#28302,#28303);
#24457=AXIS2_PLACEMENT_3D('',#35795,#28304,#28305);
#24458=AXIS2_PLACEMENT_3D('',#35804,#28310,#28311);
#24459=AXIS2_PLACEMENT_3D('',#35806,#28312,#28313);
#24460=AXIS2_PLACEMENT_3D('',#35808,#28315,#28316);
#24461=AXIS2_PLACEMENT_3D('',#35812,#28319,#28320);
#24462=AXIS2_PLACEMENT_3D('',#35813,#28321,#28322);
#24463=AXIS2_PLACEMENT_3D('',#35814,#28323,#28324);
#24464=AXIS2_PLACEMENT_3D('',#35823,#28329,#28330);
#24465=AXIS2_PLACEMENT_3D('',#35825,#28331,#28332);
#24466=AXIS2_PLACEMENT_3D('',#35827,#28334,#28335);
#24467=AXIS2_PLACEMENT_3D('',#35831,#28338,#28339);
#24468=AXIS2_PLACEMENT_3D('',#35832,#28340,#28341);
#24469=AXIS2_PLACEMENT_3D('',#35833,#28342,#28343);
#24470=AXIS2_PLACEMENT_3D('',#35842,#28348,#28349);
#24471=AXIS2_PLACEMENT_3D('',#35844,#28350,#28351);
#24472=AXIS2_PLACEMENT_3D('',#35846,#28353,#28354);
#24473=AXIS2_PLACEMENT_3D('',#35850,#28357,#28358);
#24474=AXIS2_PLACEMENT_3D('',#35851,#28359,#28360);
#24475=AXIS2_PLACEMENT_3D('',#35852,#28361,#28362);
#24476=AXIS2_PLACEMENT_3D('',#35861,#28367,#28368);
#24477=AXIS2_PLACEMENT_3D('',#35863,#28369,#28370);
#24478=AXIS2_PLACEMENT_3D('',#35865,#28372,#28373);
#24479=AXIS2_PLACEMENT_3D('',#35869,#28376,#28377);
#24480=AXIS2_PLACEMENT_3D('',#35870,#28378,#28379);
#24481=AXIS2_PLACEMENT_3D('',#35871,#28380,#28381);
#24482=AXIS2_PLACEMENT_3D('',#35880,#28386,#28387);
#24483=AXIS2_PLACEMENT_3D('',#35882,#28388,#28389);
#24484=AXIS2_PLACEMENT_3D('',#35884,#28391,#28392);
#24485=AXIS2_PLACEMENT_3D('',#35888,#28395,#28396);
#24486=AXIS2_PLACEMENT_3D('',#35889,#28397,#28398);
#24487=AXIS2_PLACEMENT_3D('',#35890,#28399,#28400);
#24488=AXIS2_PLACEMENT_3D('',#35899,#28405,#28406);
#24489=AXIS2_PLACEMENT_3D('',#35901,#28407,#28408);
#24490=AXIS2_PLACEMENT_3D('',#35903,#28410,#28411);
#24491=AXIS2_PLACEMENT_3D('',#35907,#28414,#28415);
#24492=AXIS2_PLACEMENT_3D('',#35908,#28416,#28417);
#24493=AXIS2_PLACEMENT_3D('',#35909,#28418,#28419);
#24494=AXIS2_PLACEMENT_3D('',#35918,#28424,#28425);
#24495=AXIS2_PLACEMENT_3D('',#35920,#28426,#28427);
#24496=AXIS2_PLACEMENT_3D('',#35922,#28429,#28430);
#24497=AXIS2_PLACEMENT_3D('',#35926,#28433,#28434);
#24498=AXIS2_PLACEMENT_3D('',#35927,#28435,#28436);
#24499=AXIS2_PLACEMENT_3D('',#35928,#28437,#28438);
#24500=AXIS2_PLACEMENT_3D('',#35930,#28439,#28440);
#24501=AXIS2_PLACEMENT_3D('',#35933,#28442,#28443);
#24502=AXIS2_PLACEMENT_3D('',#35934,#28444,#28445);
#24503=AXIS2_PLACEMENT_3D('',#35936,#28446,#28447);
#24504=AXIS2_PLACEMENT_3D('',#35939,#28449,#28450);
#24505=AXIS2_PLACEMENT_3D('',#35940,#28451,#28452);
#24506=AXIS2_PLACEMENT_3D('',#35941,#28453,#28454);
#24507=AXIS2_PLACEMENT_3D('',#35943,#28455,#28456);
#24508=AXIS2_PLACEMENT_3D('',#35944,#28457,#28458);
#24509=AXIS2_PLACEMENT_3D('',#35945,#28459,#28460);
#24510=AXIS2_PLACEMENT_3D('',#35947,#28461,#28462);
#24511=AXIS2_PLACEMENT_3D('',#35949,#28464,#28465);
#24512=AXIS2_PLACEMENT_3D('',#35951,#28467,#28468);
#24513=AXIS2_PLACEMENT_3D('',#35953,#28469,#28470);
#24514=AXIS2_PLACEMENT_3D('',#35954,#28471,#28472);
#24515=AXIS2_PLACEMENT_3D('',#35956,#28473,#28474);
#24516=AXIS2_PLACEMENT_3D('',#35959,#28477,#28478);
#24517=AXIS2_PLACEMENT_3D('',#35961,#28479,#28480);
#24518=AXIS2_PLACEMENT_3D('',#35962,#28481,#28482);
#24519=AXIS2_PLACEMENT_3D('',#35964,#28483,#28484);
#24520=AXIS2_PLACEMENT_3D('',#35966,#28486,#28487);
#28057=DIRECTION('axis',(0.,0.,1.));
#28058=DIRECTION('refdir',(1.,0.,0.));
#28059=DIRECTION('center_axis',(0.,6.92018220157531E-16,-1.));
#28060=DIRECTION('ref_axis',(-1.,-3.00652077147108E-17,0.));
#28061=DIRECTION('center_axis',(0.,0.,-1.));
#28062=DIRECTION('ref_axis',(-1.,-6.12323399573677E-17,0.));
#28063=DIRECTION('center_axis',(0.,0.,-1.));
#28064=DIRECTION('ref_axis',(-1.,-6.12323399573677E-17,0.));
#28065=DIRECTION('',(0.382683432365084,6.97712130664731E-16,-0.923879532511289));
#28066=DIRECTION('center_axis',(0.,0.,1.));
#28067=DIRECTION('ref_axis',(-1.,0.,0.));
#28068=DIRECTION('center_axis',(0.,0.,1.));
#28069=DIRECTION('ref_axis',(-1.,0.,0.));
#28070=DIRECTION('center_axis',(0.,0.,1.));
#28071=DIRECTION('ref_axis',(1.,0.,0.));
#28072=DIRECTION('',(0.,0.,-1.));
#28073=DIRECTION('center_axis',(0.,0.,-1.));
#28074=DIRECTION('ref_axis',(-1.,0.,0.));
#28075=DIRECTION('center_axis',(0.,0.,-1.));
#28076=DIRECTION('ref_axis',(-1.,0.,0.));
#28077=DIRECTION('center_axis',(0.,0.,-1.));
#28078=DIRECTION('ref_axis',(1.,0.,0.));
#28079=DIRECTION('center_axis',(0.,0.,1.));
#28080=DIRECTION('ref_axis',(1.,0.,0.));
#28081=DIRECTION('',(-0.707106781186548,-8.65956056235493E-17,-0.707106781186548));
#28082=DIRECTION('center_axis',(0.,0.,1.));
#28083=DIRECTION('ref_axis',(-1.,0.,0.));
#28084=DIRECTION('',(-0.707106781186545,-8.6595605623549E-17,-0.70710678118655));
#28085=DIRECTION('center_axis',(0.,0.,1.));
#28086=DIRECTION('ref_axis',(-1.,0.,0.));
#28087=DIRECTION('center_axis',(0.,0.,-1.));
#28088=DIRECTION('ref_axis',(-1.,0.,0.));
#28089=DIRECTION('center_axis',(0.,0.,1.));
#28090=DIRECTION('ref_axis',(1.,0.,0.));
#28091=DIRECTION('center_axis',(-0.714953656968427,-0.69917184467588,0.));
#28092=DIRECTION('ref_axis',(0.69917184467588,-0.714953656968427,0.));
#28093=DIRECTION('',(0.,0.,1.));
#28094=DIRECTION('',(0.69917184467588,-0.714953656968427,0.));
#28095=DIRECTION('',(0.,0.,1.));
#28096=DIRECTION('',(0.69917184467588,-0.714953656968427,0.));
#28097=DIRECTION('center_axis',(0.,0.,1.));
#28098=DIRECTION('ref_axis',(0.939692620785908,-0.342020143325669,0.));
#28099=DIRECTION('center_axis',(0.,0.,1.));
#28100=DIRECTION('ref_axis',(1.,0.,0.));
#28101=DIRECTION('',(-0.995160058598588,-0.0982672772089165,0.));
#28102=DIRECTION('center_axis',(-0.0982672772089165,0.995160058598588,0.));
#28103=DIRECTION('ref_axis',(-0.995160058598588,-0.0982672772089165,0.));
#28104=DIRECTION('',(0.,0.,-1.));
#28105=DIRECTION('',(-0.995160058598588,-0.0982672772089165,0.));
#28106=DIRECTION('center_axis',(0.,0.,1.));
#28107=DIRECTION('ref_axis',(0.939692620785908,-0.342020143325669,0.));
#28108=DIRECTION('center_axis',(0.,0.,-1.));
#28109=DIRECTION('ref_axis',(1.,0.,0.));
#28110=DIRECTION('center_axis',(-0.910967530182447,-0.412478070875644,0.));
#28111=DIRECTION('ref_axis',(0.412478070875644,-0.910967530182447,0.));
#28112=DIRECTION('',(0.,0.,1.));
#28113=DIRECTION('',(0.412478070875644,-0.910967530182447,0.));
#28114=DIRECTION('',(0.,0.,1.));
#28115=DIRECTION('',(0.412478070875644,-0.910967530182447,0.));
#28116=DIRECTION('center_axis',(0.,0.,1.));
#28117=DIRECTION('ref_axis',(0.766044443118978,-0.64278760968654,0.));
#28118=DIRECTION('center_axis',(0.,0.,1.));
#28119=DIRECTION('ref_axis',(1.,0.,0.));
#28120=DIRECTION('',(-0.968753951801183,0.248023750615928,0.));
#28121=DIRECTION('center_axis',(0.248023750615928,0.968753951801183,0.));
#28122=DIRECTION('ref_axis',(-0.968753951801183,0.248023750615928,0.));
#28123=DIRECTION('',(0.,0.,-1.));
#28124=DIRECTION('',(-0.968753951801183,0.248023750615928,0.));
#28125=DIRECTION('center_axis',(0.,0.,1.));
#28126=DIRECTION('ref_axis',(0.766044443118978,-0.64278760968654,0.));
#28127=DIRECTION('center_axis',(0.,0.,-1.));
#28128=DIRECTION('ref_axis',(1.,0.,0.));
#28129=DIRECTION('center_axis',(-0.997105274807593,-0.076033354199819,0.));
#28130=DIRECTION('ref_axis',(0.076033354199819,-0.997105274807593,0.));
#28131=DIRECTION('',(0.,0.,1.));
#28132=DIRECTION('',(0.076033354199819,-0.997105274807593,0.));
#28133=DIRECTION('',(0.,0.,1.));
#28134=DIRECTION('',(0.076033354199819,-0.997105274807593,0.));
#28135=DIRECTION('center_axis',(0.,0.,1.));
#28136=DIRECTION('ref_axis',(0.5,-0.866025403784439,0.));
#28137=DIRECTION('center_axis',(0.,0.,1.));
#28138=DIRECTION('ref_axis',(1.,0.,0.));
#28139=DIRECTION('',(-0.82550182113093,0.56439945367578,0.));
#28140=DIRECTION('center_axis',(0.56439945367578,0.82550182113093,0.));
#28141=DIRECTION('ref_axis',(-0.82550182113093,0.56439945367578,0.));
#28142=DIRECTION('',(0.,0.,-1.));
#28143=DIRECTION('',(-0.82550182113093,0.56439945367578,0.));
#28144=DIRECTION('center_axis',(0.,0.,1.));
#28145=DIRECTION('ref_axis',(0.5,-0.866025403784439,0.));
#28146=DIRECTION('center_axis',(0.,0.,-1.));
#28147=DIRECTION('ref_axis',(1.,0.,0.));
#28148=DIRECTION('center_axis',(-0.962977407584354,0.269582107125302,0.));
#28149=DIRECTION('ref_axis',(-0.269582107125302,-0.962977407584354,0.));
#28150=DIRECTION('',(0.,0.,1.));
#28151=DIRECTION('',(-0.269582107125302,-0.962977407584354,0.));
#28152=DIRECTION('',(0.,0.,1.));
#28153=DIRECTION('',(-0.269582107125302,-0.962977407584354,0.));
#28154=DIRECTION('center_axis',(0.,0.,1.));
#28155=DIRECTION('ref_axis',(0.17364817766693,-0.984807753012208,0.));
#28156=DIRECTION('center_axis',(0.,0.,1.));
#28157=DIRECTION('ref_axis',(1.,0.,0.));
#28158=DIRECTION('',(-0.582681987722944,0.81270025297353,0.));
#28159=DIRECTION('center_axis',(0.81270025297353,0.582681987722944,0.));
#28160=DIRECTION('ref_axis',(-0.582681987722944,0.81270025297353,0.));
#28161=DIRECTION('',(0.,0.,-1.));
#28162=DIRECTION('',(-0.582681987722944,0.81270025297353,0.));
#28163=DIRECTION('center_axis',(0.,0.,1.));
#28164=DIRECTION('ref_axis',(0.17364817766693,-0.984807753012208,0.));
#28165=DIRECTION('center_axis',(0.,0.,-1.));
#28166=DIRECTION('ref_axis',(1.,0.,0.));
#28167=DIRECTION('center_axis',(-0.81270025297353,0.582681987722944,0.));
#28168=DIRECTION('ref_axis',(-0.582681987722944,-0.81270025297353,0.));
#28169=DIRECTION('',(0.,0.,1.));
#28170=DIRECTION('',(-0.582681987722944,-0.81270025297353,0.));
#28171=DIRECTION('',(0.,0.,1.));
#28172=DIRECTION('',(-0.582681987722944,-0.81270025297353,0.));
#28173=DIRECTION('center_axis',(0.,0.,1.));
#28174=DIRECTION('ref_axis',(-0.17364817766693,-0.984807753012208,0.));
#28175=DIRECTION('center_axis',(0.,0.,1.));
#28176=DIRECTION('ref_axis',(1.,0.,0.));
#28177=DIRECTION('',(-0.269582107125302,0.962977407584353,0.));
#28178=DIRECTION('center_axis',(0.962977407584354,0.269582107125302,0.));
#28179=DIRECTION('ref_axis',(-0.269582107125302,0.962977407584353,0.));
#28180=DIRECTION('',(0.,0.,-1.));
#28181=DIRECTION('',(-0.269582107125302,0.962977407584353,0.));
#28182=DIRECTION('center_axis',(0.,0.,1.));
#28183=DIRECTION('ref_axis',(-0.17364817766693,-0.984807753012208,0.));
#28184=DIRECTION('center_axis',(0.,0.,-1.));
#28185=DIRECTION('ref_axis',(1.,0.,0.));
#28186=DIRECTION('center_axis',(-0.564399453675779,0.82550182113093,0.));
#28187=DIRECTION('ref_axis',(-0.82550182113093,-0.564399453675779,0.));
#28188=DIRECTION('',(0.,0.,1.));
#28189=DIRECTION('',(-0.82550182113093,-0.564399453675779,0.));
#28190=DIRECTION('',(0.,0.,1.));
#28191=DIRECTION('',(-0.82550182113093,-0.564399453675779,0.));
#28192=DIRECTION('center_axis',(0.,0.,1.));
#28193=DIRECTION('ref_axis',(-0.5,-0.866025403784438,0.));
#28194=DIRECTION('center_axis',(0.,0.,1.));
#28195=DIRECTION('ref_axis',(1.,0.,0.));
#28196=DIRECTION('',(0.0760333541998194,0.997105274807593,0.));
#28197=DIRECTION('center_axis',(0.997105274807593,-0.0760333541998194,0.));
#28198=DIRECTION('ref_axis',(0.0760333541998194,0.997105274807593,0.));
#28199=DIRECTION('',(0.,0.,-1.));
#28200=DIRECTION('',(0.0760333541998194,0.997105274807593,0.));
#28201=DIRECTION('center_axis',(0.,0.,1.));
#28202=DIRECTION('ref_axis',(-0.5,-0.866025403784438,0.));
#28203=DIRECTION('center_axis',(0.,0.,-1.));
#28204=DIRECTION('ref_axis',(1.,0.,0.));
#28205=DIRECTION('center_axis',(-0.248023750615927,0.968753951801183,0.));
#28206=DIRECTION('ref_axis',(-0.968753951801183,-0.248023750615927,0.));
#28207=DIRECTION('',(0.,0.,1.));
#28208=DIRECTION('',(-0.968753951801183,-0.248023750615927,0.));
#28209=DIRECTION('',(0.,0.,1.));
#28210=DIRECTION('',(-0.968753951801183,-0.248023750615927,0.));
#28211=DIRECTION('center_axis',(0.,0.,1.));
#28212=DIRECTION('ref_axis',(-0.766044443118978,-0.642787609686539,0.));
#28213=DIRECTION('center_axis',(0.,0.,1.));
#28214=DIRECTION('ref_axis',(1.,0.,0.));
#28215=DIRECTION('',(0.412478070875644,0.910967530182447,0.));
#28216=DIRECTION('center_axis',(0.910967530182447,-0.412478070875644,0.));
#28217=DIRECTION('ref_axis',(0.412478070875644,0.910967530182447,0.));
#28218=DIRECTION('',(0.,0.,-1.));
#28219=DIRECTION('',(0.412478070875644,0.910967530182447,0.));
#28220=DIRECTION('center_axis',(0.,0.,1.));
#28221=DIRECTION('ref_axis',(-0.766044443118978,-0.642787609686539,0.));
#28222=DIRECTION('center_axis',(0.,0.,-1.));
#28223=DIRECTION('ref_axis',(1.,0.,0.));
#28224=DIRECTION('center_axis',(0.0982672772089174,0.995160058598588,0.));
#28225=DIRECTION('ref_axis',(-0.995160058598588,0.0982672772089174,0.));
#28226=DIRECTION('',(0.,0.,1.));
#28227=DIRECTION('',(-0.995160058598588,0.0982672772089174,0.));
#28228=DIRECTION('',(0.,0.,1.));
#28229=DIRECTION('',(-0.995160058598588,0.0982672772089174,0.));
#28230=DIRECTION('center_axis',(0.,0.,1.));
#28231=DIRECTION('ref_axis',(-0.939692620785908,-0.342020143325669,0.));
#28232=DIRECTION('center_axis',(0.,0.,1.));
#28233=DIRECTION('ref_axis',(1.,0.,0.));
#28234=DIRECTION('',(0.699171844675881,0.714953656968426,0.));
#28235=DIRECTION('center_axis',(0.714953656968426,-0.699171844675881,0.));
#28236=DIRECTION('ref_axis',(0.699171844675881,0.714953656968426,0.));
#28237=DIRECTION('',(0.,0.,-1.));
#28238=DIRECTION('',(0.699171844675881,0.714953656968426,0.));
#28239=DIRECTION('center_axis',(0.,0.,1.));
#28240=DIRECTION('ref_axis',(-0.939692620785908,-0.342020143325669,0.));
#28241=DIRECTION('center_axis',(0.,0.,-1.));
#28242=DIRECTION('ref_axis',(1.,0.,0.));
#28243=DIRECTION('center_axis',(0.432705821131813,0.901535175330749,0.));
#28244=DIRECTION('ref_axis',(-0.901535175330748,0.432705821131813,0.));
#28245=DIRECTION('',(0.,0.,1.));
#28246=DIRECTION('',(-0.901535175330748,0.432705821131813,0.));
#28247=DIRECTION('',(0.,0.,1.));
#28248=DIRECTION('',(-0.901535175330748,0.432705821131813,0.));
#28249=DIRECTION('center_axis',(0.,0.,1.));
#28250=DIRECTION('ref_axis',(-1.,5.55111512312578E-17,0.));
#28251=DIRECTION('center_axis',(0.,0.,1.));
#28252=DIRECTION('ref_axis',(1.,0.,0.));
#28253=DIRECTION('',(0.901535175330749,0.432705821131813,0.));
#28254=DIRECTION('center_axis',(0.,0.,1.));
#28255=DIRECTION('ref_axis',(1.,0.,0.));
#28256=DIRECTION('center_axis',(0.432705821131813,-0.901535175330749,0.));
#28257=DIRECTION('ref_axis',(0.901535175330749,0.432705821131813,0.));
#28258=DIRECTION('',(0.,0.,-1.));
#28259=DIRECTION('',(0.901535175330749,0.432705821131813,0.));
#28260=DIRECTION('center_axis',(0.,0.,1.));
#28261=DIRECTION('ref_axis',(-1.,5.55111512312578E-17,0.));
#28262=DIRECTION('center_axis',(0.,0.,-1.));
#28263=DIRECTION('ref_axis',(1.,0.,0.));
#28264=DIRECTION('center_axis',(0.,0.,-1.));
#28265=DIRECTION('ref_axis',(1.,0.,0.));
#28266=DIRECTION('center_axis',(0.714953656968426,0.699171844675881,0.));
#28267=DIRECTION('ref_axis',(-0.699171844675881,0.714953656968426,0.));
#28268=DIRECTION('',(0.,0.,1.));
#28269=DIRECTION('',(-0.699171844675881,0.714953656968426,0.));
#28270=DIRECTION('',(0.,0.,1.));
#28271=DIRECTION('',(-0.699171844675881,0.714953656968426,0.));
#28272=DIRECTION('center_axis',(0.,0.,1.));
#28273=DIRECTION('ref_axis',(-0.939692620785908,0.342020143325669,0.));
#28274=DIRECTION('center_axis',(0.,0.,1.));
#28275=DIRECTION('ref_axis',(1.,0.,0.));
#28276=DIRECTION('',(0.995160058598588,0.0982672772089171,0.));
#28277=DIRECTION('center_axis',(0.0982672772089171,-0.995160058598588,0.));
#28278=DIRECTION('ref_axis',(0.995160058598588,0.0982672772089171,0.));
#28279=DIRECTION('',(0.,0.,-1.));
#28280=DIRECTION('',(0.995160058598588,0.0982672772089171,0.));
#28281=DIRECTION('center_axis',(0.,0.,1.));
#28282=DIRECTION('ref_axis',(-0.939692620785908,0.342020143325669,0.));
#28283=DIRECTION('center_axis',(0.,0.,-1.));
#28284=DIRECTION('ref_axis',(1.,0.,0.));
#28285=DIRECTION('center_axis',(0.910967530182447,0.412478070875644,0.));
#28286=DIRECTION('ref_axis',(-0.412478070875644,0.910967530182447,0.));
#28287=DIRECTION('',(0.,0.,1.));
#28288=DIRECTION('',(-0.412478070875644,0.910967530182447,0.));
#28289=DIRECTION('',(0.,0.,1.));
#28290=DIRECTION('',(-0.412478070875644,0.910967530182447,0.));
#28291=DIRECTION('center_axis',(0.,0.,1.));
#28292=DIRECTION('ref_axis',(-0.766044443118978,0.642787609686539,0.));
#28293=DIRECTION('center_axis',(0.,0.,1.));
#28294=DIRECTION('ref_axis',(1.,0.,0.));
#28295=DIRECTION('',(0.968753951801183,-0.248023750615928,0.));
#28296=DIRECTION('center_axis',(-0.248023750615928,-0.968753951801183,0.));
#28297=DIRECTION('ref_axis',(0.968753951801183,-0.248023750615928,0.));
#28298=DIRECTION('',(0.,0.,-1.));
#28299=DIRECTION('',(0.968753951801183,-0.248023750615928,0.));
#28300=DIRECTION('center_axis',(0.,0.,1.));
#28301=DIRECTION('ref_axis',(-0.766044443118978,0.642787609686539,0.));
#28302=DIRECTION('center_axis',(0.,0.,-1.));
#28303=DIRECTION('ref_axis',(1.,0.,0.));
#28304=DIRECTION('center_axis',(0.997105274807593,0.0760333541998187,0.));
#28305=DIRECTION('ref_axis',(-0.0760333541998187,0.997105274807593,0.));
#28306=DIRECTION('',(0.,0.,1.));
#28307=DIRECTION('',(-0.0760333541998187,0.997105274807593,0.));
#28308=DIRECTION('',(0.,0.,1.));
#28309=DIRECTION('',(-0.0760333541998187,0.997105274807593,0.));
#28310=DIRECTION('center_axis',(0.,0.,1.));
#28311=DIRECTION('ref_axis',(-0.5,0.866025403784439,0.));
#28312=DIRECTION('center_axis',(0.,0.,1.));
#28313=DIRECTION('ref_axis',(1.,0.,0.));
#28314=DIRECTION('',(0.82550182113093,-0.56439945367578,0.));
#28315=DIRECTION('center_axis',(-0.56439945367578,-0.82550182113093,0.));
#28316=DIRECTION('ref_axis',(0.82550182113093,-0.56439945367578,0.));
#28317=DIRECTION('',(0.,0.,-1.));
#28318=DIRECTION('',(0.82550182113093,-0.56439945367578,0.));
#28319=DIRECTION('center_axis',(0.,0.,1.));
#28320=DIRECTION('ref_axis',(-0.5,0.866025403784439,0.));
#28321=DIRECTION('center_axis',(0.,0.,-1.));
#28322=DIRECTION('ref_axis',(1.,0.,0.));
#28323=DIRECTION('center_axis',(0.962977407584354,-0.269582107125302,0.));
#28324=DIRECTION('ref_axis',(0.269582107125302,0.962977407584354,0.));
#28325=DIRECTION('',(0.,0.,1.));
#28326=DIRECTION('',(0.269582107125302,0.962977407584354,0.));
#28327=DIRECTION('',(0.,0.,1.));
#28328=DIRECTION('',(0.269582107125302,0.962977407584354,0.));
#28329=DIRECTION('center_axis',(0.,0.,1.));
#28330=DIRECTION('ref_axis',(-0.17364817766693,0.984807753012208,0.));
#28331=DIRECTION('center_axis',(0.,0.,1.));
#28332=DIRECTION('ref_axis',(1.,0.,0.));
#28333=DIRECTION('',(0.582681987722944,-0.81270025297353,0.));
#28334=DIRECTION('center_axis',(-0.81270025297353,-0.582681987722944,0.));
#28335=DIRECTION('ref_axis',(0.582681987722944,-0.81270025297353,0.));
#28336=DIRECTION('',(0.,0.,-1.));
#28337=DIRECTION('',(0.582681987722944,-0.81270025297353,0.));
#28338=DIRECTION('center_axis',(0.,0.,1.));
#28339=DIRECTION('ref_axis',(-0.17364817766693,0.984807753012208,0.));
#28340=DIRECTION('center_axis',(0.,0.,-1.));
#28341=DIRECTION('ref_axis',(1.,0.,0.));
#28342=DIRECTION('center_axis',(0.812700252973529,-0.582681987722944,0.));
#28343=DIRECTION('ref_axis',(0.582681987722944,0.812700252973529,0.));
#28344=DIRECTION('',(0.,0.,1.));
#28345=DIRECTION('',(0.582681987722944,0.812700252973529,0.));
#28346=DIRECTION('',(0.,0.,1.));
#28347=DIRECTION('',(0.582681987722944,0.812700252973529,0.));
#28348=DIRECTION('center_axis',(0.,0.,1.));
#28349=DIRECTION('ref_axis',(0.17364817766693,0.984807753012208,0.));
#28350=DIRECTION('center_axis',(0.,0.,1.));
#28351=DIRECTION('ref_axis',(1.,0.,0.));
#28352=DIRECTION('',(0.269582107125302,-0.962977407584354,0.));
#28353=DIRECTION('center_axis',(-0.962977407584354,-0.269582107125302,0.));
#28354=DIRECTION('ref_axis',(0.269582107125302,-0.962977407584354,0.));
#28355=DIRECTION('',(0.,0.,-1.));
#28356=DIRECTION('',(0.269582107125302,-0.962977407584354,0.));
#28357=DIRECTION('center_axis',(0.,0.,1.));
#28358=DIRECTION('ref_axis',(0.17364817766693,0.984807753012208,0.));
#28359=DIRECTION('center_axis',(0.,0.,-1.));
#28360=DIRECTION('ref_axis',(1.,0.,0.));
#28361=DIRECTION('center_axis',(0.56439945367578,-0.82550182113093,0.));
#28362=DIRECTION('ref_axis',(0.82550182113093,0.56439945367578,0.));
#28363=DIRECTION('',(0.,0.,1.));
#28364=DIRECTION('',(0.82550182113093,0.56439945367578,0.));
#28365=DIRECTION('',(0.,0.,1.));
#28366=DIRECTION('',(0.82550182113093,0.56439945367578,0.));
#28367=DIRECTION('center_axis',(0.,0.,1.));
#28368=DIRECTION('ref_axis',(0.5,0.866025403784439,0.));
#28369=DIRECTION('center_axis',(0.,0.,1.));
#28370=DIRECTION('ref_axis',(1.,0.,0.));
#28371=DIRECTION('',(-0.076033354199819,-0.997105274807593,0.));
#28372=DIRECTION('center_axis',(-0.997105274807593,0.076033354199819,0.));
#28373=DIRECTION('ref_axis',(-0.076033354199819,-0.997105274807593,0.));
#28374=DIRECTION('',(0.,0.,-1.));
#28375=DIRECTION('',(-0.076033354199819,-0.997105274807593,0.));
#28376=DIRECTION('center_axis',(0.,0.,1.));
#28377=DIRECTION('ref_axis',(0.5,0.866025403784439,0.));
#28378=DIRECTION('center_axis',(0.,0.,-1.));
#28379=DIRECTION('ref_axis',(1.,0.,0.));
#28380=DIRECTION('center_axis',(0.248023750615927,-0.968753951801183,0.));
#28381=DIRECTION('ref_axis',(0.968753951801183,0.248023750615927,0.));
#28382=DIRECTION('',(0.,0.,1.));
#28383=DIRECTION('',(0.968753951801183,0.248023750615927,0.));
#28384=DIRECTION('',(0.,0.,1.));
#28385=DIRECTION('',(0.968753951801183,0.248023750615927,0.));
#28386=DIRECTION('center_axis',(0.,0.,1.));
#28387=DIRECTION('ref_axis',(0.766044443118978,0.642787609686539,0.));
#28388=DIRECTION('center_axis',(0.,0.,1.));
#28389=DIRECTION('ref_axis',(1.,0.,0.));
#28390=DIRECTION('',(-0.412478070875644,-0.910967530182447,0.));
#28391=DIRECTION('center_axis',(-0.910967530182447,0.412478070875644,0.));
#28392=DIRECTION('ref_axis',(-0.412478070875644,-0.910967530182447,0.));
#28393=DIRECTION('',(0.,0.,-1.));
#28394=DIRECTION('',(-0.412478070875644,-0.910967530182447,0.));
#28395=DIRECTION('center_axis',(0.,0.,1.));
#28396=DIRECTION('ref_axis',(0.766044443118978,0.642787609686539,0.));
#28397=DIRECTION('center_axis',(0.,0.,-1.));
#28398=DIRECTION('ref_axis',(1.,0.,0.));
#28399=DIRECTION('center_axis',(-0.0982672772089173,-0.995160058598588,
0.));
#28400=DIRECTION('ref_axis',(0.995160058598588,-0.0982672772089173,0.));
#28401=DIRECTION('',(0.,0.,1.));
#28402=DIRECTION('',(0.995160058598588,-0.0982672772089173,0.));
#28403=DIRECTION('',(0.,0.,1.));
#28404=DIRECTION('',(0.995160058598588,-0.0982672772089173,0.));
#28405=DIRECTION('center_axis',(0.,0.,1.));
#28406=DIRECTION('ref_axis',(0.939692620785908,0.342020143325669,0.));
#28407=DIRECTION('center_axis',(0.,0.,1.));
#28408=DIRECTION('ref_axis',(1.,0.,0.));
#28409=DIRECTION('',(-0.699171844675881,-0.714953656968426,0.));
#28410=DIRECTION('center_axis',(-0.714953656968426,0.699171844675881,0.));
#28411=DIRECTION('ref_axis',(-0.699171844675881,-0.714953656968426,0.));
#28412=DIRECTION('',(0.,0.,-1.));
#28413=DIRECTION('',(-0.699171844675881,-0.714953656968426,0.));
#28414=DIRECTION('center_axis',(0.,0.,1.));
#28415=DIRECTION('ref_axis',(0.939692620785908,0.342020143325669,0.));
#28416=DIRECTION('center_axis',(0.,0.,-1.));
#28417=DIRECTION('ref_axis',(1.,0.,0.));
#28418=DIRECTION('center_axis',(-0.432705821131813,-0.901535175330749,0.));
#28419=DIRECTION('ref_axis',(0.901535175330749,-0.432705821131813,0.));
#28420=DIRECTION('',(0.,0.,1.));
#28421=DIRECTION('',(0.901535175330749,-0.432705821131813,0.));
#28422=DIRECTION('',(0.,0.,1.));
#28423=DIRECTION('',(0.901535175330749,-0.432705821131813,0.));
#28424=DIRECTION('center_axis',(0.,0.,1.));
#28425=DIRECTION('ref_axis',(1.,0.,0.));
#28426=DIRECTION('center_axis',(0.,0.,1.));
#28427=DIRECTION('ref_axis',(1.,0.,0.));
#28428=DIRECTION('',(-0.901535175330749,-0.432705821131813,0.));
#28429=DIRECTION('center_axis',(-0.432705821131813,0.901535175330749,0.));
#28430=DIRECTION('ref_axis',(-0.901535175330749,-0.432705821131813,0.));
#28431=DIRECTION('',(0.,0.,-1.));
#28432=DIRECTION('',(-0.901535175330749,-0.432705821131813,0.));
#28433=DIRECTION('center_axis',(0.,0.,1.));
#28434=DIRECTION('ref_axis',(1.,0.,0.));
#28435=DIRECTION('center_axis',(0.,0.,-1.));
#28436=DIRECTION('ref_axis',(1.,0.,0.));
#28437=DIRECTION('center_axis',(0.,0.,1.));
#28438=DIRECTION('ref_axis',(1.,0.,0.));
#28439=DIRECTION('center_axis',(0.,0.,-1.));
#28440=DIRECTION('ref_axis',(1.,0.,0.));
#28441=DIRECTION('',(0.,0.,1.));
#28442=DIRECTION('center_axis',(0.,0.,1.));
#28443=DIRECTION('ref_axis',(1.,0.,0.));
#28444=DIRECTION('center_axis',(0.,0.,1.));
#28445=DIRECTION('ref_axis',(1.,0.,0.));
#28446=DIRECTION('center_axis',(0.,0.,1.));
#28447=DIRECTION('ref_axis',(1.,0.,0.));
#28448=DIRECTION('',(0.,0.,1.));
#28449=DIRECTION('center_axis',(0.,0.,1.));
#28450=DIRECTION('ref_axis',(1.,0.,0.));
#28451=DIRECTION('center_axis',(0.,0.,1.));
#28452=DIRECTION('ref_axis',(1.,0.,0.));
#28453=DIRECTION('center_axis',(0.,0.,-1.));
#28454=DIRECTION('ref_axis',(-1.,0.,0.));
#28455=DIRECTION('center_axis',(0.,0.,1.));
#28456=DIRECTION('ref_axis',(1.,0.,0.));
#28457=DIRECTION('center_axis',(0.,0.,-1.));
#28458=DIRECTION('ref_axis',(-1.,0.,0.));
#28459=DIRECTION('center_axis',(0.,0.,1.));
#28460=DIRECTION('ref_axis',(1.,0.,0.));
#28461=DIRECTION('center_axis',(0.,0.,1.));
#28462=DIRECTION('ref_axis',(1.,0.,0.));
#28463=DIRECTION('',(0.707106781186548,8.65956056235494E-17,-0.707106781186547));
#28464=DIRECTION('center_axis',(0.,0.,1.));
#28465=DIRECTION('ref_axis',(1.,0.,0.));
#28466=DIRECTION('',(0.,0.,-1.));
#28467=DIRECTION('center_axis',(0.,0.,1.));
#28468=DIRECTION('ref_axis',(1.,0.,0.));
#28469=DIRECTION('center_axis',(0.,0.,1.));
#28470=DIRECTION('ref_axis',(1.,0.,0.));
#28471=DIRECTION('center_axis',(0.,0.,1.));
#28472=DIRECTION('ref_axis',(1.,0.,0.));
#28473=DIRECTION('center_axis',(0.,0.,1.));
#28474=DIRECTION('ref_axis',(1.,0.,0.));
#28475=DIRECTION('',(0.,0.,-1.));
#28476=DIRECTION('',(0.,0.,-1.));
#28477=DIRECTION('center_axis',(0.,0.,1.));
#28478=DIRECTION('ref_axis',(1.,0.,0.));
#28479=DIRECTION('center_axis',(0.,0.,1.));
#28480=DIRECTION('ref_axis',(1.,0.,0.));
#28481=DIRECTION('center_axis',(0.,0.,1.));
#28482=DIRECTION('ref_axis',(1.,0.,0.));
#28483=DIRECTION('center_axis',(0.,0.,1.));
#28484=DIRECTION('ref_axis',(1.,0.,0.));
#28485=DIRECTION('',(0.,0.,-1.));
#28486=DIRECTION('center_axis',(0.,0.,1.));
#28487=DIRECTION('ref_axis',(1.,0.,0.));
#35554=CARTESIAN_POINT('',(0.,0.,0.));
#35555=CARTESIAN_POINT('Origin',(0.,-1.77202349450337E-17,5.1056066017178));
#35556=CARTESIAN_POINT('',(0.578786796564404,-7.08809397801347E-17,5.1312132034356));
#35557=CARTESIAN_POINT('',(-0.578786796564404,-7.08809397801347E-17,5.1312132034356));
#35558=CARTESIAN_POINT('Origin',(0.,-3.54404698900674E-17,5.1312132034356));
#35559=CARTESIAN_POINT('Origin',(0.,-3.54404698900674E-17,5.1312132034356));
#35560=CARTESIAN_POINT('',(0.6,7.34788079488412E-17,5.08));
#35561=CARTESIAN_POINT('',(0.589393398282202,7.2179873864488E-17,5.1056066017178));
#35562=CARTESIAN_POINT('',(-0.6,-7.34788079488412E-17,5.08));
#35563=CARTESIAN_POINT('Origin',(0.,0.,5.08));
#35564=CARTESIAN_POINT('Origin',(0.,0.,5.08));
#35565=CARTESIAN_POINT('Origin',(0.,0.,4.93));
#35566=CARTESIAN_POINT('',(-0.6,-7.34788079488412E-17,4.78));
#35567=CARTESIAN_POINT('',(-0.6,-7.34788079488412E-17,4.93));
#35568=CARTESIAN_POINT('',(0.6,-7.34788079488412E-17,4.78));
#35569=CARTESIAN_POINT('Origin',(0.,0.,4.78));
#35570=CARTESIAN_POINT('Origin',(0.,0.,4.78));
#35571=CARTESIAN_POINT('Origin',(0.,0.,5.13));
#35572=CARTESIAN_POINT('',(-0.56,-6.85802207522518E-17,5.15));
#35573=CARTESIAN_POINT('Origin',(0.,0.,5.15));
#35574=CARTESIAN_POINT('',(-0.58,-7.10295143505465E-17,5.13));
#35575=CARTESIAN_POINT('Origin',(0.,0.,4.765));
#35576=CARTESIAN_POINT('',(0.57,6.98048675513991E-17,4.75));
#35577=CARTESIAN_POINT('',(0.585,7.16418377501202E-17,4.765));
#35578=CARTESIAN_POINT('Origin',(0.,0.,4.75));
#35579=CARTESIAN_POINT('Origin',(0.6,0.,4.75));
#35580=CARTESIAN_POINT('',(-0.4,-4.89858719658941E-17,4.75));
#35581=CARTESIAN_POINT('Origin',(0.,0.,4.75));
#35582=CARTESIAN_POINT('Origin',(0.263113933820054,-0.0957656401311874,
5.25));
#35583=CARTESIAN_POINT('',(0.278507289184601,-0.111506456633887,5.25));
#35584=CARTESIAN_POINT('',(0.278507289184601,-0.111506456633887,5.75));
#35585=CARTESIAN_POINT('',(0.278507289184601,-0.111506456633887,5.475));
#35586=CARTESIAN_POINT('',(0.263113933820054,-0.0957656401311874,5.25));
#35587=CARTESIAN_POINT('',(0.263113933820054,-0.0957656401311874,5.25));
#35588=CARTESIAN_POINT('',(0.263113933820054,-0.0957656401311874,5.75));
#35589=CARTESIAN_POINT('',(0.263113933820054,-0.0957656401311874,5.25));
#35590=CARTESIAN_POINT('',(0.263113933820054,-0.0957656401311874,5.75));
#35591=CARTESIAN_POINT('Origin',(0.291304712443632,-0.106026244430958,5.75));
#35592=CARTESIAN_POINT('',(0.285023929972306,-0.0936021332189712,5.75));
#35593=CARTESIAN_POINT('Origin',(0.,0.,5.75));
#35594=CARTESIAN_POINT('',(0.329344964122349,-0.0892256439182034,5.75));
#35595=CARTESIAN_POINT('Origin',(0.329344964122349,-0.0892256439182034,
5.25));
#35596=CARTESIAN_POINT('',(0.285023929972306,-0.0936021332189712,5.25));
#35597=CARTESIAN_POINT('',(0.285023929972306,-0.0936021332189712,5.475));
#35598=CARTESIAN_POINT('',(0.329344964122349,-0.0892256439182034,5.25));
#35599=CARTESIAN_POINT('Origin',(0.291304712443632,-0.106026244430958,5.25));
#35600=CARTESIAN_POINT('Origin',(0.,0.,5.25));
#35601=CARTESIAN_POINT('Origin',(0.214492444073314,-0.179980530712231,5.25));
#35602=CARTESIAN_POINT('',(0.223573790202197,-0.200036897433009,5.25));
#35603=CARTESIAN_POINT('',(0.223573790202197,-0.200036897433009,5.75));
#35604=CARTESIAN_POINT('',(0.223573790202197,-0.200036897433009,5.475));
#35605=CARTESIAN_POINT('',(0.214492444073314,-0.179980530712231,5.25));
#35606=CARTESIAN_POINT('',(0.214492444073314,-0.179980530712231,5.25));
#35607=CARTESIAN_POINT('',(0.214492444073314,-0.179980530712231,5.75));
#35608=CARTESIAN_POINT('',(0.214492444073314,-0.179980530712231,5.25));
#35609=CARTESIAN_POINT('',(0.214492444073314,-0.179980530712231,5.75));
#35610=CARTESIAN_POINT('Origin',(0.237473777366883,-0.199264159002827,5.75));
#35611=CARTESIAN_POINT('',(0.235821068723235,-0.18544115925606,5.75));
#35612=CARTESIAN_POINT('Origin',(0.,0.,5.75));
#35613=CARTESIAN_POINT('',(0.278966064957542,-0.19648729100752,5.75));
#35614=CARTESIAN_POINT('Origin',(0.278966064957542,-0.19648729100752,5.25));
#35615=CARTESIAN_POINT('',(0.235821068723235,-0.18544115925606,5.25));
#35616=CARTESIAN_POINT('',(0.235821068723235,-0.18544115925606,5.475));
#35617=CARTESIAN_POINT('',(0.278966064957542,-0.19648729100752,5.25));
#35618=CARTESIAN_POINT('Origin',(0.237473777366883,-0.199264159002827,5.25));
#35619=CARTESIAN_POINT('Origin',(0.,0.,5.25));
#35620=CARTESIAN_POINT('Origin',(0.14,-0.242487113059643,5.25));
#35621=CARTESIAN_POINT('',(0.141673992523682,-0.264439936171524,5.25));
#35622=CARTESIAN_POINT('',(0.141673992523682,-0.264439936171524,5.75));
#35623=CARTESIAN_POINT('',(0.141673992523682,-0.264439936171524,5.475));
#35624=CARTESIAN_POINT('',(0.14,-0.242487113059643,5.25));
#35625=CARTESIAN_POINT('',(0.14,-0.242487113059643,5.25));
#35626=CARTESIAN_POINT('',(0.14,-0.242487113059643,5.75));
#35627=CARTESIAN_POINT('',(0.14,-0.242487113059643,5.25));
#35628=CARTESIAN_POINT('',(0.14,-0.242487113059643,5.75));
#35629=CARTESIAN_POINT('Origin',(0.155,-0.268467875173176,5.75));
#35630=CARTESIAN_POINT('',(0.158174706237834,-0.254913244666837,5.75));
#35631=CARTESIAN_POINT('Origin',(0.,0.,5.75));
#35632=CARTESIAN_POINT('',(0.194939741258221,-0.280049670957756,5.75));
#35633=CARTESIAN_POINT('Origin',(0.194939741258221,-0.280049670957756,5.25));
#35634=CARTESIAN_POINT('',(0.158174706237834,-0.254913244666837,5.25));
#35635=CARTESIAN_POINT('',(0.158174706237834,-0.254913244666837,5.475));
#35636=CARTESIAN_POINT('',(0.194939741258221,-0.280049670957756,5.25));
#35637=CARTESIAN_POINT('Origin',(0.155,-0.268467875173176,5.25));
#35638=CARTESIAN_POINT('Origin',(0.,0.,5.25));
#35639=CARTESIAN_POINT('Origin',(0.0486214897467404,-0.275746170843418,
5.25));
#35640=CARTESIAN_POINT('',(0.0426862204613663,-0.296947615889947,5.25));
#35641=CARTESIAN_POINT('',(0.0426862204613663,-0.296947615889947,5.75));
#35642=CARTESIAN_POINT('',(0.0426862204613663,-0.296947615889947,5.475));
#35643=CARTESIAN_POINT('',(0.0486214897467404,-0.275746170843418,5.25));
#35644=CARTESIAN_POINT('',(0.0486214897467404,-0.275746170843418,5.25));
#35645=CARTESIAN_POINT('',(0.0486214897467404,-0.275746170843418,5.75));
#35646=CARTESIAN_POINT('',(0.0486214897467404,-0.275746170843418,5.25));
#35647=CARTESIAN_POINT('',(0.0486214897467404,-0.275746170843418,5.75));
#35648=CARTESIAN_POINT('Origin',(0.0538309350767483,-0.305290403433784,
5.75));
#35649=CARTESIAN_POINT('',(0.0614501397701088,-0.293639030651979,5.75));
#35650=CARTESIAN_POINT('Origin',(0.,0.,5.75));
#35651=CARTESIAN_POINT('',(0.0874008077589859,-0.32983392749753,5.75));
#35652=CARTESIAN_POINT('Origin',(0.0874008077589859,-0.32983392749753,5.25));
#35653=CARTESIAN_POINT('',(0.0614501397701088,-0.293639030651979,5.25));
#35654=CARTESIAN_POINT('',(0.0614501397701088,-0.293639030651979,5.475));
#35655=CARTESIAN_POINT('',(0.0874008077589859,-0.32983392749753,5.25));
#35656=CARTESIAN_POINT('Origin',(0.0538309350767483,-0.305290403433784,
5.25));
#35657=CARTESIAN_POINT('Origin',(0.,0.,5.25));
#35658=CARTESIAN_POINT('Origin',(-0.0486214897467405,-0.275746170843418,
5.25));
#35659=CARTESIAN_POINT('',(-0.0614501397701088,-0.293639030651979,5.25));
#35660=CARTESIAN_POINT('',(-0.0614501397701088,-0.293639030651979,5.75));
#35661=CARTESIAN_POINT('',(-0.0614501397701088,-0.293639030651979,5.475));
#35662=CARTESIAN_POINT('',(-0.0486214897467405,-0.275746170843418,5.25));
#35663=CARTESIAN_POINT('',(-0.0486214897467405,-0.275746170843418,5.25));
#35664=CARTESIAN_POINT('',(-0.0486214897467405,-0.275746170843418,5.75));
#35665=CARTESIAN_POINT('',(-0.0486214897467405,-0.275746170843418,5.25));
#35666=CARTESIAN_POINT('',(-0.0486214897467405,-0.275746170843418,5.75));
#35667=CARTESIAN_POINT('Origin',(-0.0538309350767484,-0.305290403433785,
5.75));
#35668=CARTESIAN_POINT('',(-0.0426862204613664,-0.296947615889947,5.75));
#35669=CARTESIAN_POINT('Origin',(0.,0.,5.75));
#35670=CARTESIAN_POINT('',(-0.0306799530545266,-0.339835344550771,5.75));
#35671=CARTESIAN_POINT('Origin',(-0.0306799530545266,-0.339835344550771,
5.25));
#35672=CARTESIAN_POINT('',(-0.0426862204613664,-0.296947615889947,5.25));
#35673=CARTESIAN_POINT('',(-0.0426862204613664,-0.296947615889947,5.475));
#35674=CARTESIAN_POINT('',(-0.0306799530545266,-0.339835344550771,5.25));
#35675=CARTESIAN_POINT('Origin',(-0.0538309350767484,-0.305290403433785,
5.25));
#35676=CARTESIAN_POINT('Origin',(0.,0.,5.25));
#35677=CARTESIAN_POINT('Origin',(-0.14,-0.242487113059643,5.25));
#35678=CARTESIAN_POINT('',(-0.158174706237835,-0.254913244666837,5.25));
#35679=CARTESIAN_POINT('',(-0.158174706237835,-0.254913244666837,5.75));
#35680=CARTESIAN_POINT('',(-0.158174706237835,-0.254913244666837,5.475));
#35681=CARTESIAN_POINT('',(-0.14,-0.242487113059643,5.25));
#35682=CARTESIAN_POINT('',(-0.14,-0.242487113059643,5.25));
#35683=CARTESIAN_POINT('',(-0.14,-0.242487113059643,5.75));
#35684=CARTESIAN_POINT('',(-0.14,-0.242487113059643,5.25));
#35685=CARTESIAN_POINT('',(-0.14,-0.242487113059643,5.75));
#35686=CARTESIAN_POINT('Origin',(-0.155,-0.268467875173176,5.75));
#35687=CARTESIAN_POINT('',(-0.141673992523682,-0.264439936171524,5.75));
#35688=CARTESIAN_POINT('Origin',(0.,0.,5.75));
#35689=CARTESIAN_POINT('',(-0.14506025874178,-0.308847603615662,5.75));
#35690=CARTESIAN_POINT('Origin',(-0.14506025874178,-0.308847603615662,5.25));
#35691=CARTESIAN_POINT('',(-0.141673992523682,-0.264439936171524,5.25));
#35692=CARTESIAN_POINT('',(-0.141673992523682,-0.264439936171524,5.475));
#35693=CARTESIAN_POINT('',(-0.14506025874178,-0.308847603615662,5.25));
#35694=CARTESIAN_POINT('Origin',(-0.155,-0.268467875173176,5.25));
#35695=CARTESIAN_POINT('Origin',(0.,0.,5.25));
#35696=CARTESIAN_POINT('Origin',(-0.214492444073314,-0.179980530712231,
5.25));
#35697=CARTESIAN_POINT('',(-0.235821068723235,-0.18544115925606,5.25));
#35698=CARTESIAN_POINT('',(-0.235821068723235,-0.18544115925606,5.75));
#35699=CARTESIAN_POINT('',(-0.235821068723235,-0.18544115925606,5.475));
#35700=CARTESIAN_POINT('',(-0.214492444073314,-0.179980530712231,5.25));
#35701=CARTESIAN_POINT('',(-0.214492444073314,-0.179980530712231,5.25));
#35702=CARTESIAN_POINT('',(-0.214492444073314,-0.179980530712231,5.75));
#35703=CARTESIAN_POINT('',(-0.214492444073314,-0.179980530712231,5.25));
#35704=CARTESIAN_POINT('',(-0.214492444073314,-0.179980530712231,5.75));
#35705=CARTESIAN_POINT('Origin',(-0.237473777366883,-0.199264159002827,
5.75));
#35706=CARTESIAN_POINT('',(-0.223573790202197,-0.200036897433008,5.75));
#35707=CARTESIAN_POINT('Origin',(0.,0.,5.75));
#35708=CARTESIAN_POINT('',(-0.241944156363363,-0.240608283579327,5.75));
#35709=CARTESIAN_POINT('Origin',(-0.241944156363363,-0.240608283579327,
5.25));
#35710=CARTESIAN_POINT('',(-0.223573790202197,-0.200036897433008,5.25));
#35711=CARTESIAN_POINT('',(-0.223573790202197,-0.200036897433008,5.475));
#35712=CARTESIAN_POINT('',(-0.241944156363363,-0.240608283579327,5.25));
#35713=CARTESIAN_POINT('Origin',(-0.237473777366883,-0.199264159002827,
5.25));
#35714=CARTESIAN_POINT('Origin',(0.,0.,5.25));
#35715=CARTESIAN_POINT('Origin',(-0.263113933820054,-0.0957656401311872,
5.25));
#35716=CARTESIAN_POINT('',(-0.285023929972306,-0.0936021332189709,5.25));
#35717=CARTESIAN_POINT('',(-0.285023929972306,-0.0936021332189709,5.75));
#35718=CARTESIAN_POINT('',(-0.285023929972306,-0.0936021332189709,5.475));
#35719=CARTESIAN_POINT('',(-0.263113933820054,-0.0957656401311872,5.25));
#35720=CARTESIAN_POINT('',(-0.263113933820054,-0.0957656401311872,5.25));
#35721=CARTESIAN_POINT('',(-0.263113933820054,-0.0957656401311872,5.75));
#35722=CARTESIAN_POINT('',(-0.263113933820054,-0.0957656401311872,5.25));
#35723=CARTESIAN_POINT('',(-0.263113933820054,-0.0957656401311872,5.75));
#35724=CARTESIAN_POINT('Origin',(-0.291304712443632,-0.106026244430957,
5.75));
#35725=CARTESIAN_POINT('',(-0.278507289184601,-0.111506456633887,5.75));
#35726=CARTESIAN_POINT('Origin',(0.,0.,5.75));
#35727=CARTESIAN_POINT('',(-0.309646018012069,-0.143348053543252,5.75));
#35728=CARTESIAN_POINT('Origin',(-0.309646018012069,-0.143348053543252,
5.25));
#35729=CARTESIAN_POINT('',(-0.278507289184601,-0.111506456633887,5.25));
#35730=CARTESIAN_POINT('',(-0.278507289184601,-0.111506456633887,5.475));
#35731=CARTESIAN_POINT('',(-0.309646018012069,-0.143348053543252,5.25));
#35732=CARTESIAN_POINT('Origin',(-0.291304712443632,-0.106026244430957,
5.25));
#35733=CARTESIAN_POINT('Origin',(0.,0.,5.25));
#35734=CARTESIAN_POINT('Origin',(-0.28,1.38777878078145E-17,5.25));
#35735=CARTESIAN_POINT('',(-0.299848698761516,0.00952669150468696,5.25));
#35736=CARTESIAN_POINT('',(-0.299848698761516,0.00952669150468696,5.75));
#35737=CARTESIAN_POINT('',(-0.299848698761516,0.00952669150468698,5.475));
#35738=CARTESIAN_POINT('',(-0.28,1.38777878078145E-17,5.25));
#35739=CARTESIAN_POINT('',(-0.28,1.38777878078145E-17,5.25));
#35740=CARTESIAN_POINT('',(-0.28,1.38777878078145E-17,5.75));
#35741=CARTESIAN_POINT('',(-0.28,1.38777878078145E-17,5.25));
#35742=CARTESIAN_POINT('',(-0.28,1.38777878078145E-17,5.75));
#35743=CARTESIAN_POINT('Origin',(-0.31,2.77555756156289E-17,5.75));
#35744=CARTESIAN_POINT('',(-0.3,-3.67394039744206E-17,5.75));
#35745=CARTESIAN_POINT('Origin',(0.,0.,5.75));
#35746=CARTESIAN_POINT('',(-0.299848698761516,-0.00952669150468687,5.75));
#35747=CARTESIAN_POINT('',(-0.34,-0.0287979326579064,5.75));
#35748=CARTESIAN_POINT('Origin',(0.,0.,5.75));
#35749=CARTESIAN_POINT('Origin',(-0.34,-0.0287979326579064,5.25));
#35750=CARTESIAN_POINT('',(-0.299848698761516,-0.00952669150468687,5.25));
#35751=CARTESIAN_POINT('',(-0.299848698761516,-0.00952669150468689,5.475));
#35752=CARTESIAN_POINT('',(-0.34,-0.0287979326579064,5.25));
#35753=CARTESIAN_POINT('Origin',(-0.31,2.77555756156289E-17,5.25));
#35754=CARTESIAN_POINT('',(-0.3,-3.67394039744206E-17,5.25));
#35755=CARTESIAN_POINT('Origin',(0.,0.,5.25));
#35756=CARTESIAN_POINT('Origin',(0.,0.,5.25));
#35757=CARTESIAN_POINT('Origin',(-0.263113933820054,0.0957656401311873,
5.25));
#35758=CARTESIAN_POINT('',(-0.278507289184601,0.111506456633887,5.25));
#35759=CARTESIAN_POINT('',(-0.278507289184601,0.111506456633887,5.75));
#35760=CARTESIAN_POINT('',(-0.278507289184601,0.111506456633887,5.475));
#35761=CARTESIAN_POINT('',(-0.263113933820054,0.0957656401311873,5.25));
#35762=CARTESIAN_POINT('',(-0.263113933820054,0.0957656401311873,5.25));
#35763=CARTESIAN_POINT('',(-0.263113933820054,0.0957656401311873,5.75));
#35764=CARTESIAN_POINT('',(-0.263113933820054,0.0957656401311873,5.25));
#35765=CARTESIAN_POINT('',(-0.263113933820054,0.0957656401311873,5.75));
#35766=CARTESIAN_POINT('Origin',(-0.291304712443632,0.106026244430957,5.75));
#35767=CARTESIAN_POINT('',(-0.285023929972306,0.093602133218971,5.75));
#35768=CARTESIAN_POINT('Origin',(0.,0.,5.75));
#35769=CARTESIAN_POINT('',(-0.329344964122349,0.0892256439182032,5.75));
#35770=CARTESIAN_POINT('Origin',(-0.329344964122349,0.0892256439182032,
5.25));
#35771=CARTESIAN_POINT('',(-0.285023929972306,0.093602133218971,5.25));
#35772=CARTESIAN_POINT('',(-0.285023929972306,0.093602133218971,5.475));
#35773=CARTESIAN_POINT('',(-0.329344964122349,0.0892256439182032,5.25));
#35774=CARTESIAN_POINT('Origin',(-0.291304712443632,0.106026244430957,5.25));
#35775=CARTESIAN_POINT('Origin',(0.,0.,5.25));
#35776=CARTESIAN_POINT('Origin',(-0.214492444073314,0.179980530712231,5.25));
#35777=CARTESIAN_POINT('',(-0.223573790202197,0.200036897433008,5.25));
#35778=CARTESIAN_POINT('',(-0.223573790202197,0.200036897433008,5.75));
#35779=CARTESIAN_POINT('',(-0.223573790202197,0.200036897433008,5.475));
#35780=CARTESIAN_POINT('',(-0.214492444073314,0.179980530712231,5.25));
#35781=CARTESIAN_POINT('',(-0.214492444073314,0.179980530712231,5.25));
#35782=CARTESIAN_POINT('',(-0.214492444073314,0.179980530712231,5.75));
#35783=CARTESIAN_POINT('',(-0.214492444073314,0.179980530712231,5.25));
#35784=CARTESIAN_POINT('',(-0.214492444073314,0.179980530712231,5.75));
#35785=CARTESIAN_POINT('Origin',(-0.237473777366883,0.199264159002827,5.75));
#35786=CARTESIAN_POINT('',(-0.235821068723235,0.18544115925606,5.75));
#35787=CARTESIAN_POINT('Origin',(0.,0.,5.75));
#35788=CARTESIAN_POINT('',(-0.278966064957542,0.19648729100752,5.75));
#35789=CARTESIAN_POINT('Origin',(-0.278966064957542,0.19648729100752,5.25));
#35790=CARTESIAN_POINT('',(-0.235821068723235,0.18544115925606,5.25));
#35791=CARTESIAN_POINT('',(-0.235821068723235,0.18544115925606,5.475));
#35792=CARTESIAN_POINT('',(-0.278966064957542,0.19648729100752,5.25));
#35793=CARTESIAN_POINT('Origin',(-0.237473777366883,0.199264159002827,5.25));
#35794=CARTESIAN_POINT('Origin',(0.,0.,5.25));
#35795=CARTESIAN_POINT('Origin',(-0.14,0.242487113059643,5.25));
#35796=CARTESIAN_POINT('',(-0.141673992523682,0.264439936171524,5.25));
#35797=CARTESIAN_POINT('',(-0.141673992523682,0.264439936171524,5.75));
#35798=CARTESIAN_POINT('',(-0.141673992523682,0.264439936171524,5.475));
#35799=CARTESIAN_POINT('',(-0.14,0.242487113059643,5.25));
#35800=CARTESIAN_POINT('',(-0.14,0.242487113059643,5.25));
#35801=CARTESIAN_POINT('',(-0.14,0.242487113059643,5.75));
#35802=CARTESIAN_POINT('',(-0.14,0.242487113059643,5.25));
#35803=CARTESIAN_POINT('',(-0.14,0.242487113059643,5.75));
#35804=CARTESIAN_POINT('Origin',(-0.155,0.268467875173176,5.75));
#35805=CARTESIAN_POINT('',(-0.158174706237834,0.254913244666837,5.75));
#35806=CARTESIAN_POINT('Origin',(0.,0.,5.75));
#35807=CARTESIAN_POINT('',(-0.19493974125822,0.280049670957756,5.75));
#35808=CARTESIAN_POINT('Origin',(-0.19493974125822,0.280049670957756,5.25));
#35809=CARTESIAN_POINT('',(-0.158174706237834,0.254913244666837,5.25));
#35810=CARTESIAN_POINT('',(-0.158174706237834,0.254913244666837,5.475));
#35811=CARTESIAN_POINT('',(-0.19493974125822,0.280049670957756,5.25));
#35812=CARTESIAN_POINT('Origin',(-0.155,0.268467875173176,5.25));
#35813=CARTESIAN_POINT('Origin',(0.,0.,5.25));
#35814=CARTESIAN_POINT('Origin',(-0.0486214897467405,0.275746170843418,
5.25));
#35815=CARTESIAN_POINT('',(-0.0426862204613664,0.296947615889947,5.25));
#35816=CARTESIAN_POINT('',(-0.0426862204613664,0.296947615889947,5.75));
#35817=CARTESIAN_POINT('',(-0.0426862204613664,0.296947615889947,5.475));
#35818=CARTESIAN_POINT('',(-0.0486214897467405,0.275746170843418,5.25));
#35819=CARTESIAN_POINT('',(-0.0486214897467405,0.275746170843418,5.25));
#35820=CARTESIAN_POINT('',(-0.0486214897467405,0.275746170843418,5.75));
#35821=CARTESIAN_POINT('',(-0.0486214897467405,0.275746170843418,5.25));
#35822=CARTESIAN_POINT('',(-0.0486214897467405,0.275746170843418,5.75));
#35823=CARTESIAN_POINT('Origin',(-0.0538309350767484,0.305290403433784,
5.75));
#35824=CARTESIAN_POINT('',(-0.0614501397701089,0.293639030651979,5.75));
#35825=CARTESIAN_POINT('Origin',(0.,0.,5.75));
#35826=CARTESIAN_POINT('',(-0.0874008077589861,0.32983392749753,5.75));
#35827=CARTESIAN_POINT('Origin',(-0.0874008077589861,0.32983392749753,5.25));
#35828=CARTESIAN_POINT('',(-0.0614501397701089,0.293639030651979,5.25));
#35829=CARTESIAN_POINT('',(-0.0614501397701089,0.293639030651979,5.475));
#35830=CARTESIAN_POINT('',(-0.0874008077589861,0.32983392749753,5.25));
#35831=CARTESIAN_POINT('Origin',(-0.0538309350767484,0.305290403433784,
5.25));
#35832=CARTESIAN_POINT('Origin',(0.,0.,5.25));
#35833=CARTESIAN_POINT('Origin',(0.0486214897467405,0.275746170843418,5.25));
#35834=CARTESIAN_POINT('',(0.0614501397701089,0.293639030651979,5.25));
#35835=CARTESIAN_POINT('',(0.0614501397701089,0.293639030651979,5.75));
#35836=CARTESIAN_POINT('',(0.0614501397701089,0.293639030651979,5.475));
#35837=CARTESIAN_POINT('',(0.0486214897467405,0.275746170843418,5.25));
#35838=CARTESIAN_POINT('',(0.0486214897467405,0.275746170843418,5.25));
#35839=CARTESIAN_POINT('',(0.0486214897467405,0.275746170843418,5.75));
#35840=CARTESIAN_POINT('',(0.0486214897467405,0.275746170843418,5.25));
#35841=CARTESIAN_POINT('',(0.0486214897467405,0.275746170843418,5.75));
#35842=CARTESIAN_POINT('Origin',(0.0538309350767484,0.305290403433784,5.75));
#35843=CARTESIAN_POINT('',(0.0426862204613665,0.296947615889947,5.75));
#35844=CARTESIAN_POINT('Origin',(0.,0.,5.75));
#35845=CARTESIAN_POINT('',(0.0306799530545266,0.339835344550771,5.75));
#35846=CARTESIAN_POINT('Origin',(0.0306799530545266,0.339835344550771,5.25));
#35847=CARTESIAN_POINT('',(0.0426862204613665,0.296947615889947,5.25));
#35848=CARTESIAN_POINT('',(0.0426862204613665,0.296947615889947,5.475));
#35849=CARTESIAN_POINT('',(0.0306799530545266,0.339835344550771,5.25));
#35850=CARTESIAN_POINT('Origin',(0.0538309350767484,0.305290403433784,5.25));
#35851=CARTESIAN_POINT('Origin',(0.,0.,5.25));
#35852=CARTESIAN_POINT('Origin',(0.14,0.242487113059643,5.25));
#35853=CARTESIAN_POINT('',(0.158174706237834,0.254913244666837,5.25));
#35854=CARTESIAN_POINT('',(0.158174706237834,0.254913244666837,5.75));
#35855=CARTESIAN_POINT('',(0.158174706237834,0.254913244666837,5.475));
#35856=CARTESIAN_POINT('',(0.14,0.242487113059643,5.25));
#35857=CARTESIAN_POINT('',(0.14,0.242487113059643,5.25));
#35858=CARTESIAN_POINT('',(0.14,0.242487113059643,5.75));
#35859=CARTESIAN_POINT('',(0.14,0.242487113059643,5.25));
#35860=CARTESIAN_POINT('',(0.14,0.242487113059643,5.75));
#35861=CARTESIAN_POINT('Origin',(0.155,0.268467875173176,5.75));
#35862=CARTESIAN_POINT('',(0.141673992523682,0.264439936171524,5.75));
#35863=CARTESIAN_POINT('Origin',(0.,0.,5.75));
#35864=CARTESIAN_POINT('',(0.14506025874178,0.308847603615662,5.75));
#35865=CARTESIAN_POINT('Origin',(0.14506025874178,0.308847603615662,5.25));
#35866=CARTESIAN_POINT('',(0.141673992523682,0.264439936171524,5.25));
#35867=CARTESIAN_POINT('',(0.141673992523682,0.264439936171524,5.475));
#35868=CARTESIAN_POINT('',(0.14506025874178,0.308847603615662,5.25));
#35869=CARTESIAN_POINT('Origin',(0.155,0.268467875173176,5.25));
#35870=CARTESIAN_POINT('Origin',(0.,0.,5.25));
#35871=CARTESIAN_POINT('Origin',(0.214492444073314,0.179980530712231,5.25));
#35872=CARTESIAN_POINT('',(0.235821068723235,0.18544115925606,5.25));
#35873=CARTESIAN_POINT('',(0.235821068723235,0.18544115925606,5.75));
#35874=CARTESIAN_POINT('',(0.235821068723235,0.18544115925606,5.475));
#35875=CARTESIAN_POINT('',(0.214492444073314,0.179980530712231,5.25));
#35876=CARTESIAN_POINT('',(0.214492444073314,0.179980530712231,5.25));
#35877=CARTESIAN_POINT('',(0.214492444073314,0.179980530712231,5.75));
#35878=CARTESIAN_POINT('',(0.214492444073314,0.179980530712231,5.25));
#35879=CARTESIAN_POINT('',(0.214492444073314,0.179980530712231,5.75));
#35880=CARTESIAN_POINT('Origin',(0.237473777366883,0.199264159002827,5.75));
#35881=CARTESIAN_POINT('',(0.223573790202197,0.200036897433008,5.75));
#35882=CARTESIAN_POINT('Origin',(0.,0.,5.75));
#35883=CARTESIAN_POINT('',(0.241944156363363,0.240608283579327,5.75));
#35884=CARTESIAN_POINT('Origin',(0.241944156363363,0.240608283579327,5.25));
#35885=CARTESIAN_POINT('',(0.223573790202197,0.200036897433008,5.25));
#35886=CARTESIAN_POINT('',(0.223573790202197,0.200036897433008,5.475));
#35887=CARTESIAN_POINT('',(0.241944156363363,0.240608283579327,5.25));
#35888=CARTESIAN_POINT('Origin',(0.237473777366883,0.199264159002827,5.25));
#35889=CARTESIAN_POINT('Origin',(0.,0.,5.25));
#35890=CARTESIAN_POINT('Origin',(0.263113933820054,0.0957656401311872,5.25));
#35891=CARTESIAN_POINT('',(0.285023929972306,0.0936021332189709,5.25));
#35892=CARTESIAN_POINT('',(0.285023929972306,0.0936021332189709,5.75));
#35893=CARTESIAN_POINT('',(0.285023929972306,0.0936021332189709,5.475));
#35894=CARTESIAN_POINT('',(0.263113933820054,0.0957656401311872,5.25));
#35895=CARTESIAN_POINT('',(0.263113933820054,0.0957656401311872,5.25));
#35896=CARTESIAN_POINT('',(0.263113933820054,0.0957656401311872,5.75));
#35897=CARTESIAN_POINT('',(0.263113933820054,0.0957656401311872,5.25));
#35898=CARTESIAN_POINT('',(0.263113933820054,0.0957656401311872,5.75));
#35899=CARTESIAN_POINT('Origin',(0.291304712443632,0.106026244430957,5.75));
#35900=CARTESIAN_POINT('',(0.278507289184601,0.111506456633887,5.75));
#35901=CARTESIAN_POINT('Origin',(0.,0.,5.75));
#35902=CARTESIAN_POINT('',(0.309646018012069,0.143348053543252,5.75));
#35903=CARTESIAN_POINT('Origin',(0.309646018012069,0.143348053543252,5.25));
#35904=CARTESIAN_POINT('',(0.278507289184601,0.111506456633887,5.25));
#35905=CARTESIAN_POINT('',(0.278507289184601,0.111506456633887,5.475));
#35906=CARTESIAN_POINT('',(0.309646018012069,0.143348053543252,5.25));
#35907=CARTESIAN_POINT('Origin',(0.291304712443632,0.106026244430957,5.25));
#35908=CARTESIAN_POINT('Origin',(0.,0.,5.25));
#35909=CARTESIAN_POINT('Origin',(0.28,0.,5.25));
#35910=CARTESIAN_POINT('',(0.299848698761516,-0.00952669150468695,5.25));
#35911=CARTESIAN_POINT('',(0.299848698761516,-0.00952669150468695,5.75));
#35912=CARTESIAN_POINT('',(0.299848698761516,-0.00952669150468696,5.475));
#35913=CARTESIAN_POINT('',(0.28,0.,5.25));
#35914=CARTESIAN_POINT('',(0.28,0.,5.25));
#35915=CARTESIAN_POINT('',(0.28,0.,5.75));
#35916=CARTESIAN_POINT('',(0.28,0.,5.25));
#35917=CARTESIAN_POINT('',(0.28,0.,5.75));
#35918=CARTESIAN_POINT('Origin',(0.31,0.,5.75));
#35919=CARTESIAN_POINT('',(0.299848698761516,0.00952669150468695,5.75));
#35920=CARTESIAN_POINT('Origin',(0.,0.,5.75));
#35921=CARTESIAN_POINT('',(0.34,0.0287979326579064,5.75));
#35922=CARTESIAN_POINT('Origin',(0.34,0.0287979326579064,5.25));
#35923=CARTESIAN_POINT('',(0.299848698761516,0.00952669150468695,5.25));
#35924=CARTESIAN_POINT('',(0.299848698761516,0.00952669150468693,5.475));
#35925=CARTESIAN_POINT('',(0.34,0.0287979326579064,5.25));
#35926=CARTESIAN_POINT('Origin',(0.31,0.,5.25));
#35927=CARTESIAN_POINT('Origin',(0.,0.,5.25));
#35928=CARTESIAN_POINT('Origin',(0.,0.,-0.005));
#35929=CARTESIAN_POINT('',(-0.24,2.93915231795365E-17,0.));
#35930=CARTESIAN_POINT('Origin',(0.,0.,0.));
#35931=CARTESIAN_POINT('',(-0.24,-2.93915231795365E-17,0.04));
#35932=CARTESIAN_POINT('',(-0.24,-2.93915231795365E-17,-0.005));
#35933=CARTESIAN_POINT('Origin',(0.,0.,0.04));
#35934=CARTESIAN_POINT('Origin',(0.,0.,-0.005));
#35935=CARTESIAN_POINT('',(-0.28,-3.42901103761259E-17,0.));
#35936=CARTESIAN_POINT('Origin',(0.,0.,0.));
#35937=CARTESIAN_POINT('',(-0.28,-3.42901103761259E-17,0.04));
#35938=CARTESIAN_POINT('',(-0.28,-3.42901103761259E-17,-0.005));
#35939=CARTESIAN_POINT('Origin',(0.,0.,0.04));
#35940=CARTESIAN_POINT('Origin',(0.24,0.,0.04));
#35941=CARTESIAN_POINT('Origin',(0.38,0.,0.));
#35942=CARTESIAN_POINT('',(-0.38,-4.65365783675994E-17,-1.05818132034585E-16));
#35943=CARTESIAN_POINT('Origin',(0.,0.,0.));
#35944=CARTESIAN_POINT('Origin',(0.38,0.,0.));
#35945=CARTESIAN_POINT('Origin',(0.,0.,0.00999999999999979));
#35946=CARTESIAN_POINT('',(-0.4,-4.89858719658941E-17,0.0199999999999997));
#35947=CARTESIAN_POINT('Origin',(0.,0.,0.0199999999999996));
#35948=CARTESIAN_POINT('',(-0.39,-4.77612251667468E-17,0.00999999999999979));
#35949=CARTESIAN_POINT('Origin',(0.,0.,2.385));
#35950=CARTESIAN_POINT('',(-0.4,-4.89858719658941E-17,2.385));
#35951=CARTESIAN_POINT('Origin',(0.3,0.,5.15));
#35952=CARTESIAN_POINT('',(-0.3,-3.67394039744206E-17,5.15));
#35953=CARTESIAN_POINT('Origin',(0.,0.,5.15));
#35954=CARTESIAN_POINT('Origin',(0.,0.,5.475));
#35955=CARTESIAN_POINT('',(-0.3,-3.67394039744206E-17,5.8));
#35956=CARTESIAN_POINT('Origin',(0.,0.,5.8));
#35957=CARTESIAN_POINT('',(-0.3,-3.67394039744206E-17,5.475));
#35958=CARTESIAN_POINT('',(-0.3,-3.67394039744206E-17,5.475));
#35959=CARTESIAN_POINT('Origin',(0.18,0.,5.8));
#35960=CARTESIAN_POINT('',(-0.18,-2.20436423846524E-17,5.8));
#35961=CARTESIAN_POINT('Origin',(0.,0.,5.8));
#35962=CARTESIAN_POINT('Origin',(0.,0.,5.95));
#35963=CARTESIAN_POINT('',(-0.18,-2.20436423846524E-17,6.1));
#35964=CARTESIAN_POINT('Origin',(0.,0.,6.1));
#35965=CARTESIAN_POINT('',(-0.18,-2.20436423846524E-17,5.95));
#35966=CARTESIAN_POINT('Origin',(0.,0.,6.1));
#53624=UNCERTAINTY_MEASURE_WITH_UNIT(LENGTH_MEASURE(0.001),#53651,
'DISTANCE_ACCURACY_VALUE',
'Maximum model space distance between geometric entities at asserted c
onnectivities');
#53632=UNCERTAINTY_MEASURE_WITH_UNIT(LENGTH_MEASURE(0.001),#53651,
'DISTANCE_ACCURACY_VALUE',
'Maximum model space distance between geometric entities at asserted c
onnectivities');
#53642=(
GEOMETRIC_REPRESENTATION_CONTEXT(3)
GLOBAL_UNCERTAINTY_ASSIGNED_CONTEXT((#53624))
GLOBAL_UNIT_ASSIGNED_CONTEXT((#53651,#53653,#53654))
REPRESENTATION_CONTEXT('','3D')
);
#53650=(
GEOMETRIC_REPRESENTATION_CONTEXT(3)
GLOBAL_UNCERTAINTY_ASSIGNED_CONTEXT((#53632))
GLOBAL_UNIT_ASSIGNED_CONTEXT((#53651,#53653,#53654))
REPRESENTATION_CONTEXT('','3D')
);
#53651=(
LENGTH_UNIT()
NAMED_UNIT(*)
SI_UNIT(.CENTI.,.METRE.)
);
#53653=(
NAMED_UNIT(*)
PLANE_ANGLE_UNIT()
SI_UNIT($,.RADIAN.)
);
#53654=(
NAMED_UNIT(*)
SI_UNIT($,.STERADIAN.)
SOLID_ANGLE_UNIT()
);
#53664=SHAPE_DEFINITION_REPRESENTATION(#53681,#53732);
#53681=PRODUCT_DEFINITION_SHAPE('',$,#53750);
#53732=SHAPE_REPRESENTATION('',(#24374),#53642);
#53740=PRODUCT_DEFINITION_CONTEXT('part definition',#53793,'design');
#53750=PRODUCT_DEFINITION('2026-10-18-22-44-41-622',
'07_Capacitive_Cavity_Gap_Sensor_D8',#53767,#53740);
#53767=PRODUCT_DEFINITION_FORMATION('',$,#53804);
#53793=APPLICATION_CONTEXT(
'Core Data for Automotive Mechanical Design Process');
#53794=PRODUCT_CONTEXT('part definition',#53793,'mechanical');
#53804=PRODUCT('2026-10-18-22-44-41-622',
'07_Capacitive_Cavity_Gap_Sensor_D8',$,(#53794));
#53938=COLOUR_RGB('Light Blue',0.38,0.62,0.78);
#53939=FILL_AREA_STYLE_COLOUR('',#53938);
#53940=FILL_AREA_STYLE('',(#53939));
#53941=SURFACE_STYLE_FILL_AREA(#53940);
#53942=SURFACE_SIDE_STYLE('',(#53941));
#53943=SURFACE_STYLE_USAGE(.BOTH.,#53942);
#53944=PRESENTATION_STYLE_ASSIGNMENT((#53943));
ENDSEC;
END-ISO-10303-21;
